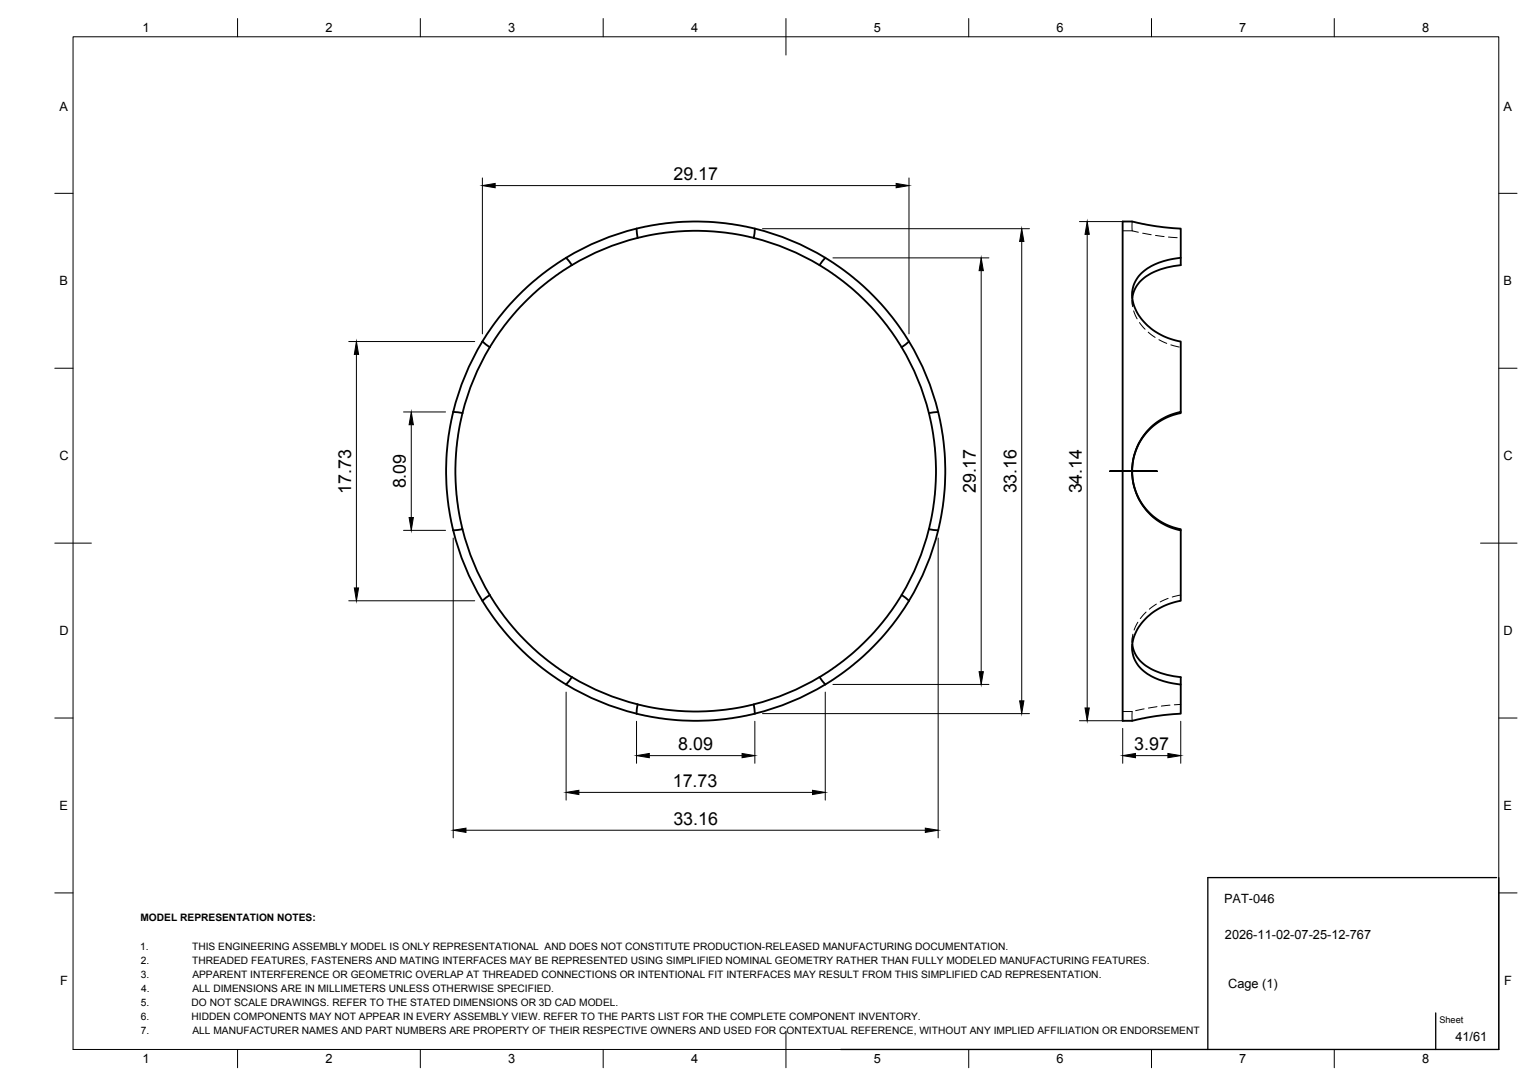
ISO-10303-21;
HEADER;
/* Generated by software containing ST-Developer
 * from STEP Tools, Inc. (www.steptools.com) 
 */

FILE_DESCRIPTION(
/* description */ ('Gear mesh backlash fixture'),
/* implementation_level */ '2;1');

FILE_NAME(
/* name */ 'Cage (1).step',
/* time_stamp */ '2026-10-28T03:26:00-07:00',
/* author */ (''),
/* organization */ (''),
/* preprocessor_version */ 'ST-DEVELOPER v20.2',
/* originating_system */ 'Autodesk Translation Framework v15.17.0.0',
/* authorisation */ '');

FILE_SCHEMA (('AUTOMOTIVE_DESIGN { 1 0 10303 214 3 1 1 }'));
ENDSEC;

DATA;
#10=MECHANICAL_DESIGN_GEOMETRIC_PRESENTATION_REPRESENTATION('',(#1061),#57900);
#751=SPHERICAL_SURFACE('',#14966,0.412776);
#752=SPHERICAL_SURFACE('',#14982,0.412776);
#753=SPHERICAL_SURFACE('',#14987,0.412776);
#754=SPHERICAL_SURFACE('',#14992,0.412776);
#755=SPHERICAL_SURFACE('',#14997,0.412776);
#756=SPHERICAL_SURFACE('',#15002,0.412776);
#757=SPHERICAL_SURFACE('',#15007,0.412776);
#758=SPHERICAL_SURFACE('',#15015,0.412776);
#809=B_SPLINE_CURVE_WITH_KNOTS('',3,(#21520,#21521,#21522,#21523,#21524,
#21525,#21526,#21527,#21528,#21529,#21530,#21531,#21532,#21533,#21534,#21535,
#21536,#21537,#21538,#21539,#21540,#21541),.UNSPECIFIED.,.F.,.F.,(4,2,2,
2,2,2,2,2,2,2,4),(0.0789094028588958,0.210573405340968,0.315860108011452,
0.421146810681936,0.522142632548711,0.623138454415485,0.72413427628226,
0.825130098149035,0.930416800819519,1.03570350349,1.16736750597208),
 .UNSPECIFIED.);
#810=B_SPLINE_CURVE_WITH_KNOTS('',3,(#21545,#21546,#21547,#21548,#21549,
#21550,#21551,#21552,#21553,#21554,#21555,#21556,#21557,#21558,#21559,#21560,
#21561,#21562,#21563,#21564,#21565,#21566),.UNSPECIFIED.,.F.,.F.,(4,2,2,
2,2,2,2,2,2,2,4),(0.0774793363974613,0.142088896491891,0.284177792983782,
0.411119756996526,0.514392970548519,0.617666184100513,0.720939397652506,
0.8242126112045,0.951154575217244,1.09324347170913,1.15785303180356),
 .UNSPECIFIED.);
#811=B_SPLINE_CURVE_WITH_KNOTS('',3,(#21572,#21573,#21574,#21575,#21576,
#21577,#21578,#21579,#21580,#21581,#21582,#21583,#21584,#21585,#21586,#21587,
#21588,#21589,#21590,#21591,#21592,#21593),.UNSPECIFIED.,.F.,.F.,(4,2,2,
2,2,2,2,2,2,2,4),(0.0774793363974613,0.142088896491891,0.284177792983782,
0.411119756996525,0.514392970548519,0.617666184100513,0.720939397652506,
0.8242126112045,0.951154575217243,1.09324347170913,1.15785303180356),
 .UNSPECIFIED.);
#812=B_SPLINE_CURVE_WITH_KNOTS('',3,(#21597,#21598,#21599,#21600,#21601,
#21602,#21603,#21604,#21605,#21606,#21607,#21608,#21609,#21610,#21611,#21612,
#21613,#21614,#21615,#21616,#21617,#21618),.UNSPECIFIED.,.F.,.F.,(4,2,2,
2,2,2,2,2,2,2,4),(0.0774793363974614,0.142088896491891,0.284177792983781,
0.411119756996525,0.514392970548519,0.617666184100512,0.720939397652506,
0.824212611204499,0.951154575217243,1.09324347170913,1.15785303180356),
 .UNSPECIFIED.);
#813=B_SPLINE_CURVE_WITH_KNOTS('',3,(#21622,#21623,#21624,#21625,#21626,
#21627,#21628,#21629,#21630,#21631,#21632,#21633),.UNSPECIFIED.,.F.,.F.,
(4,2,2,2,2,4),(0.0774793363974613,0.142088896491891,0.284177792983781,0.411119756996525,
0.514392970548519,0.617666184100512),.UNSPECIFIED.);
#814=B_SPLINE_CURVE_WITH_KNOTS('',3,(#21638,#21639,#21640,#21641,#21642,
#21643,#21644,#21645,#21646,#21647,#21648,#21649),.UNSPECIFIED.,.F.,.F.,
(4,2,2,2,2,4),(0.617666184100512,0.720939397652506,0.824212611204499,0.951154575217243,
1.09324347170913,1.15785303180356),.UNSPECIFIED.);
#815=B_SPLINE_CURVE_WITH_KNOTS('',3,(#21653,#21654,#21655,#21656,#21657,
#21658,#21659,#21660,#21661,#21662,#21663,#21664,#21665,#21666,#21667,#21668,
#21669,#21670,#21671,#21672,#21673,#21674),.UNSPECIFIED.,.F.,.F.,(4,2,2,
2,2,2,2,2,2,2,4),(0.0774793363974613,0.142088896491891,0.284177792983782,
0.411119756996526,0.514392970548519,0.617666184100513,0.720939397652507,
0.8242126112045,0.951154575217245,1.09324347170914,1.15785303180356),
 .UNSPECIFIED.);
#816=B_SPLINE_CURVE_WITH_KNOTS('',3,(#21678,#21679,#21680,#21681,#21682,
#21683,#21684,#21685,#21686,#21687,#21688,#21689,#21690,#21691,#21692,#21693,
#21694,#21695,#21696,#21697,#21698,#21699),.UNSPECIFIED.,.F.,.F.,(4,2,2,
2,2,2,2,2,2,2,4),(0.0774793363974613,0.142088896491891,0.284177792983782,
0.411119756996526,0.514392970548519,0.617666184100513,0.720939397652506,
0.824212611204499,0.951154575217243,1.09324347170913,1.15785303180356),
 .UNSPECIFIED.);
#817=B_SPLINE_CURVE_WITH_KNOTS('',3,(#21703,#21704,#21705,#21706,#21707,
#21708,#21709,#21710,#21711,#21712,#21713,#21714,#21715,#21716,#21717,#21718,
#21719,#21720,#21721,#21722,#21723,#21724),.UNSPECIFIED.,.F.,.F.,(4,2,2,
2,2,2,2,2,2,2,4),(0.0774793363974613,0.142088896491891,0.284177792983782,
0.411119756996526,0.514392970548519,0.617666184100513,0.720939397652506,
0.8242126112045,0.951154575217244,1.09324347170913,1.15785303180356),
 .UNSPECIFIED.);
#818=B_SPLINE_CURVE_WITH_KNOTS('',3,(#21728,#21729,#21730,#21731,#21732,
#21733,#21734,#21735,#21736,#21737,#21738,#21739,#21740,#21741,#21742,#21743,
#21744,#21745,#21746,#21747,#21748,#21749),.UNSPECIFIED.,.F.,.F.,(4,2,2,
2,2,2,2,2,2,2,4),(0.0774793363974613,0.142088896491891,0.284177792983782,
0.411119756996526,0.514392970548519,0.617666184100513,0.720939397652506,
0.8242126112045,0.951154575217243,1.09324347170913,1.15785303180356),
 .UNSPECIFIED.);
#819=B_SPLINE_CURVE_WITH_KNOTS('',3,(#21757,#21758,#21759,#21760,#21761,
#21762,#21763,#21764,#21765,#21766,#21767,#21768,#21769,#21770,#21771,#21772,
#21773,#21774,#21775,#21776,#21777,#21778),.UNSPECIFIED.,.F.,.F.,(4,2,2,
2,2,2,2,2,2,2,4),(0.0789094028588958,0.210573405340968,0.315860108011452,
0.421146810681936,0.522142632548711,0.623138454415485,0.72413427628226,
0.825130098149035,0.930416800819519,1.03570350349,1.16736750597208),
 .UNSPECIFIED.);
#820=B_SPLINE_CURVE_WITH_KNOTS('',3,(#21786,#21787,#21788,#21789,#21790,
#21791,#21792,#21793,#21794,#21795,#21796,#21797,#21798,#21799,#21800,#21801,
#21802,#21803,#21804,#21805,#21806,#21807),.UNSPECIFIED.,.F.,.F.,(4,2,2,
2,2,2,2,2,2,2,4),(0.0789094028588958,0.210573405340969,0.315860108011453,
0.421146810681937,0.522142632548712,0.623138454415486,0.724134276282261,
0.825130098149035,0.930416800819519,1.03570350349,1.16736750597208),
 .UNSPECIFIED.);
#821=B_SPLINE_CURVE_WITH_KNOTS('',3,(#21816,#21817,#21818,#21819,#21820,
#21821,#21822,#21823,#21824,#21825,#21826,#21827),.UNSPECIFIED.,.F.,.F.,
(4,2,2,2,2,4),(0.0789094028588958,0.210573405340968,0.315860108011452,0.421146810681937,
0.522142632548711,0.623138454415486),.UNSPECIFIED.);
#822=B_SPLINE_CURVE_WITH_KNOTS('',3,(#21829,#21830,#21831,#21832,#21833,
#21834,#21835,#21836,#21837,#21838,#21839,#21840),.UNSPECIFIED.,.F.,.F.,
(4,2,2,2,2,4),(0.623138454415486,0.72413427628226,0.825130098149035,0.930416800819519,
1.03570350349,1.16736750597208),.UNSPECIFIED.);
#823=B_SPLINE_CURVE_WITH_KNOTS('',3,(#21847,#21848,#21849,#21850,#21851,
#21852,#21853,#21854,#21855,#21856,#21857,#21858,#21859,#21860,#21861,#21862,
#21863,#21864,#21865,#21866,#21867,#21868),.UNSPECIFIED.,.F.,.F.,(4,2,2,
2,2,2,2,2,2,2,4),(0.0789094028588958,0.210573405340968,0.315860108011452,
0.421146810681936,0.522142632548711,0.623138454415486,0.72413427628226,
0.825130098149035,0.930416800819519,1.03570350349,1.16736750597208),
 .UNSPECIFIED.);
#824=B_SPLINE_CURVE_WITH_KNOTS('',3,(#21876,#21877,#21878,#21879,#21880,
#21881,#21882,#21883,#21884,#21885,#21886,#21887,#21888,#21889,#21890,#21891,
#21892,#21893,#21894,#21895,#21896,#21897),.UNSPECIFIED.,.F.,.F.,(4,2,2,
2,2,2,2,2,2,2,4),(0.0789094028588957,0.210573405340968,0.315860108011452,
0.421146810681936,0.522142632548711,0.623138454415485,0.72413427628226,
0.825130098149035,0.930416800819519,1.03570350349,1.16736750597207),
 .UNSPECIFIED.);
#825=B_SPLINE_CURVE_WITH_KNOTS('',3,(#21905,#21906,#21907,#21908,#21909,
#21910,#21911,#21912,#21913,#21914,#21915,#21916,#21917,#21918,#21919,#21920,
#21921,#21922,#21923,#21924,#21925,#21926),.UNSPECIFIED.,.F.,.F.,(4,2,2,
2,2,2,2,2,2,2,4),(0.0789094028588958,0.210573405340968,0.315860108011452,
0.421146810681936,0.522142632548711,0.623138454415486,0.72413427628226,
0.825130098149035,0.930416800819519,1.03570350349,1.16736750597208),
 .UNSPECIFIED.);
#826=B_SPLINE_CURVE_WITH_KNOTS('',3,(#21935,#21936,#21937,#21938,#21939,
#21940,#21941,#21942,#21943,#21944,#21945,#21946,#21947,#21948,#21949,#21950,
#21951,#21952,#21953,#21954,#21955,#21956),.UNSPECIFIED.,.F.,.F.,(4,2,2,
2,2,2,2,2,2,2,4),(0.0789094028588958,0.210573405340968,0.315860108011452,
0.421146810681936,0.522142632548711,0.623138454415485,0.72413427628226,
0.825130098149035,0.930416800819519,1.03570350349,1.16736750597208),
 .UNSPECIFIED.);
#947=SHAPE_REPRESENTATION_RELATIONSHIP('SRR','None',#58146,#997);
#997=ADVANCED_BREP_SHAPE_REPRESENTATION('',(#1124),#57879);
#1061=STYLED_ITEM('',(#58465),#1124);
#1124=MANIFOLD_SOLID_BREP('Continuous crown cage',#13623);
#1286=FACE_BOUND('',#2994,.T.);
#1536=PLANE('',#14979);
#1537=PLANE('',#14984);
#1538=PLANE('',#14989);
#1539=PLANE('',#14994);
#1540=PLANE('',#14999);
#1541=PLANE('',#15004);
#1542=PLANE('',#15013);
#1543=PLANE('',#15017);
#1544=PLANE('',#15018);
#2068=FACE_OUTER_BOUND('',#2976,.T.);
#2069=FACE_OUTER_BOUND('',#2977,.T.);
#2070=FACE_OUTER_BOUND('',#2978,.T.);
#2071=FACE_OUTER_BOUND('',#2979,.T.);
#2072=FACE_OUTER_BOUND('',#2980,.T.);
#2073=FACE_OUTER_BOUND('',#2981,.T.);
#2074=FACE_OUTER_BOUND('',#2982,.T.);
#2075=FACE_OUTER_BOUND('',#2983,.T.);
#2076=FACE_OUTER_BOUND('',#2984,.T.);
#2077=FACE_OUTER_BOUND('',#2985,.T.);
#2078=FACE_OUTER_BOUND('',#2986,.T.);
#2079=FACE_OUTER_BOUND('',#2987,.T.);
#2080=FACE_OUTER_BOUND('',#2988,.T.);
#2081=FACE_OUTER_BOUND('',#2989,.T.);
#2082=FACE_OUTER_BOUND('',#2990,.T.);
#2083=FACE_OUTER_BOUND('',#2991,.T.);
#2084=FACE_OUTER_BOUND('',#2992,.T.);
#2085=FACE_OUTER_BOUND('',#2993,.T.);
#2086=FACE_OUTER_BOUND('',#2995,.T.);
#2976=EDGE_LOOP('',(#10555,#10556,#10557,#10558));
#2977=EDGE_LOOP('',(#10559,#10560,#10561,#10562,#10563,#10564,#10565,#10566,
#10567,#10568,#10569,#10570,#10571,#10572,#10573,#10574,#10575,#10576,#10577,
#10578));
#2978=EDGE_LOOP('',(#10579,#10580,#10581,#10582));
#2979=EDGE_LOOP('',(#10583,#10584,#10585,#10586));
#2980=EDGE_LOOP('',(#10587,#10588,#10589,#10590));
#2981=EDGE_LOOP('',(#10591,#10592,#10593,#10594));
#2982=EDGE_LOOP('',(#10595,#10596,#10597,#10598));
#2983=EDGE_LOOP('',(#10599,#10600,#10601,#10602,#10603,#10604));
#2984=EDGE_LOOP('',(#10605,#10606,#10607,#10608));
#2985=EDGE_LOOP('',(#10609,#10610,#10611,#10612));
#2986=EDGE_LOOP('',(#10613,#10614,#10615,#10616));
#2987=EDGE_LOOP('',(#10617,#10618,#10619,#10620));
#2988=EDGE_LOOP('',(#10621,#10622,#10623,#10624));
#2989=EDGE_LOOP('',(#10625,#10626,#10627,#10628));
#2990=EDGE_LOOP('',(#10629,#10630,#10631,#10632,#10633,#10634,#10635,#10636,
#10637,#10638,#10639,#10640,#10641,#10642,#10643,#10644,#10645,#10646,#10647,
#10648));
#2991=EDGE_LOOP('',(#10649,#10650,#10651,#10652));
#2992=EDGE_LOOP('',(#10653,#10654,#10655,#10656));
#2993=EDGE_LOOP('',(#10657));
#2994=EDGE_LOOP('',(#10658));
#2995=EDGE_LOOP('',(#10659,#10660,#10661,#10662));
#3873=LINE('',#21635,#4762);
#3874=LINE('',#21931,#4763);
#4762=VECTOR('',#17596,1.706752);
#4763=VECTOR('',#17673,1.643248);
#5540=CIRCLE('',#14967,0.405071403305639);
#5541=CIRCLE('',#14968,0.405071403305639);
#5542=CIRCLE('',#14970,1.706752);
#5543=CIRCLE('',#14971,1.706752);
#5544=CIRCLE('',#14972,1.706752);
#5545=CIRCLE('',#14973,1.706752);
#5546=CIRCLE('',#14974,1.706752);
#5547=CIRCLE('',#14975,1.706752);
#5548=CIRCLE('',#14976,1.706752);
#5549=CIRCLE('',#14977,1.706752);
#5550=CIRCLE('',#14978,1.706752);
#5551=CIRCLE('',#14980,1.643248);
#5552=CIRCLE('',#14981,0.405071403305639);
#5553=CIRCLE('',#14983,0.405071403305639);
#5554=CIRCLE('',#14985,1.643248);
#5555=CIRCLE('',#14986,0.405071403305639);
#5556=CIRCLE('',#14988,0.405071403305639);
#5557=CIRCLE('',#14990,1.643248);
#5558=CIRCLE('',#14991,0.405071403305639);
#5559=CIRCLE('',#14993,0.405071403305639);
#5560=CIRCLE('',#14995,1.643248);
#5561=CIRCLE('',#14996,0.405071403305639);
#5562=CIRCLE('',#14998,0.405071403305639);
#5563=CIRCLE('',#15000,1.643248);
#5564=CIRCLE('',#15001,0.405071403305639);
#5565=CIRCLE('',#15003,0.405071403305639);
#5566=CIRCLE('',#15005,1.643248);
#5567=CIRCLE('',#15006,0.405071403305639);
#5568=CIRCLE('',#15008,0.405071403305639);
#5569=CIRCLE('',#15010,1.643248);
#5570=CIRCLE('',#15011,1.643248);
#5571=CIRCLE('',#15012,1.643248);
#5572=CIRCLE('',#15014,0.405071403305639);
#5573=CIRCLE('',#15016,0.405071403305639);
#6350=VERTEX_POINT('',#21518);
#6351=VERTEX_POINT('',#21519);
#6352=VERTEX_POINT('',#21542);
#6353=VERTEX_POINT('',#21544);
#6354=VERTEX_POINT('',#21569);
#6355=VERTEX_POINT('',#21571);
#6356=VERTEX_POINT('',#21594);
#6357=VERTEX_POINT('',#21596);
#6358=VERTEX_POINT('',#21619);
#6359=VERTEX_POINT('',#21621);
#6360=VERTEX_POINT('',#21634);
#6361=VERTEX_POINT('',#21637);
#6362=VERTEX_POINT('',#21650);
#6363=VERTEX_POINT('',#21652);
#6364=VERTEX_POINT('',#21675);
#6365=VERTEX_POINT('',#21677);
#6366=VERTEX_POINT('',#21700);
#6367=VERTEX_POINT('',#21702);
#6368=VERTEX_POINT('',#21725);
#6369=VERTEX_POINT('',#21727);
#6370=VERTEX_POINT('',#21752);
#6371=VERTEX_POINT('',#21756);
#6372=VERTEX_POINT('',#21781);
#6373=VERTEX_POINT('',#21785);
#6374=VERTEX_POINT('',#21810);
#6375=VERTEX_POINT('',#21814);
#6376=VERTEX_POINT('',#21815);
#6377=VERTEX_POINT('',#21842);
#6378=VERTEX_POINT('',#21846);
#6379=VERTEX_POINT('',#21871);
#6380=VERTEX_POINT('',#21875);
#6381=VERTEX_POINT('',#21900);
#6382=VERTEX_POINT('',#21904);
#6383=VERTEX_POINT('',#21929);
#6384=VERTEX_POINT('',#21932);
#6385=VERTEX_POINT('',#21934);
#7864=EDGE_CURVE('',#6350,#6351,#809,.T.);
#7865=EDGE_CURVE('',#6352,#6350,#5540,.T.);
#7866=EDGE_CURVE('',#6353,#6352,#810,.T.);
#7867=EDGE_CURVE('',#6351,#6353,#5541,.T.);
#7868=EDGE_CURVE('',#6354,#6352,#5542,.T.);
#7869=EDGE_CURVE('',#6354,#6355,#811,.T.);
#7870=EDGE_CURVE('',#6356,#6355,#5543,.T.);
#7871=EDGE_CURVE('',#6356,#6357,#812,.T.);
#7872=EDGE_CURVE('',#6358,#6357,#5544,.T.);
#7873=EDGE_CURVE('',#6358,#6359,#813,.T.);
#7874=EDGE_CURVE('',#6359,#6360,#3873,.T.);
#7875=EDGE_CURVE('',#6360,#6360,#5545,.T.);
#7876=EDGE_CURVE('',#6359,#6361,#814,.T.);
#7877=EDGE_CURVE('',#6362,#6361,#5546,.T.);
#7878=EDGE_CURVE('',#6362,#6363,#815,.T.);
#7879=EDGE_CURVE('',#6364,#6363,#5547,.T.);
#7880=EDGE_CURVE('',#6364,#6365,#816,.T.);
#7881=EDGE_CURVE('',#6366,#6365,#5548,.T.);
#7882=EDGE_CURVE('',#6366,#6367,#817,.T.);
#7883=EDGE_CURVE('',#6368,#6367,#5549,.T.);
#7884=EDGE_CURVE('',#6368,#6369,#818,.T.);
#7885=EDGE_CURVE('',#6353,#6369,#5550,.T.);
#7886=EDGE_CURVE('',#6350,#6370,#5551,.T.);
#7887=EDGE_CURVE('',#6370,#6354,#5552,.T.);
#7888=EDGE_CURVE('',#6371,#6370,#819,.T.);
#7889=EDGE_CURVE('',#6355,#6371,#5553,.T.);
#7890=EDGE_CURVE('',#6371,#6372,#5554,.T.);
#7891=EDGE_CURVE('',#6372,#6356,#5555,.T.);
#7892=EDGE_CURVE('',#6373,#6372,#820,.T.);
#7893=EDGE_CURVE('',#6357,#6373,#5556,.T.);
#7894=EDGE_CURVE('',#6373,#6374,#5557,.T.);
#7895=EDGE_CURVE('',#6374,#6358,#5558,.T.);
#7896=EDGE_CURVE('',#6375,#6376,#821,.T.);
#7897=EDGE_CURVE('',#6361,#6375,#5559,.T.);
#7898=EDGE_CURVE('',#6376,#6374,#822,.T.);
#7899=EDGE_CURVE('',#6375,#6377,#5560,.T.);
#7900=EDGE_CURVE('',#6377,#6362,#5561,.T.);
#7901=EDGE_CURVE('',#6378,#6377,#823,.T.);
#7902=EDGE_CURVE('',#6363,#6378,#5562,.T.);
#7903=EDGE_CURVE('',#6378,#6379,#5563,.T.);
#7904=EDGE_CURVE('',#6379,#6364,#5564,.T.);
#7905=EDGE_CURVE('',#6380,#6379,#824,.T.);
#7906=EDGE_CURVE('',#6365,#6380,#5565,.T.);
#7907=EDGE_CURVE('',#6380,#6381,#5566,.T.);
#7908=EDGE_CURVE('',#6381,#6366,#5567,.T.);
#7909=EDGE_CURVE('',#6382,#6381,#825,.T.);
#7910=EDGE_CURVE('',#6367,#6382,#5568,.T.);
#7911=EDGE_CURVE('',#6383,#6383,#5569,.T.);
#7912=EDGE_CURVE('',#6383,#6376,#3874,.T.);
#7913=EDGE_CURVE('',#6384,#6351,#5570,.T.);
#7914=EDGE_CURVE('',#6384,#6385,#826,.T.);
#7915=EDGE_CURVE('',#6382,#6385,#5571,.T.);
#7916=EDGE_CURVE('',#6369,#6384,#5572,.T.);
#7917=EDGE_CURVE('',#6385,#6368,#5573,.T.);
#10555=ORIENTED_EDGE('',*,*,#7864,.F.);
#10556=ORIENTED_EDGE('',*,*,#7865,.F.);
#10557=ORIENTED_EDGE('',*,*,#7866,.F.);
#10558=ORIENTED_EDGE('',*,*,#7867,.F.);
#10559=ORIENTED_EDGE('',*,*,#7866,.T.);
#10560=ORIENTED_EDGE('',*,*,#7868,.F.);
#10561=ORIENTED_EDGE('',*,*,#7869,.T.);
#10562=ORIENTED_EDGE('',*,*,#7870,.F.);
#10563=ORIENTED_EDGE('',*,*,#7871,.T.);
#10564=ORIENTED_EDGE('',*,*,#7872,.F.);
#10565=ORIENTED_EDGE('',*,*,#7873,.T.);
#10566=ORIENTED_EDGE('',*,*,#7874,.T.);
#10567=ORIENTED_EDGE('',*,*,#7875,.F.);
#10568=ORIENTED_EDGE('',*,*,#7874,.F.);
#10569=ORIENTED_EDGE('',*,*,#7876,.T.);
#10570=ORIENTED_EDGE('',*,*,#7877,.F.);
#10571=ORIENTED_EDGE('',*,*,#7878,.T.);
#10572=ORIENTED_EDGE('',*,*,#7879,.F.);
#10573=ORIENTED_EDGE('',*,*,#7880,.T.);
#10574=ORIENTED_EDGE('',*,*,#7881,.F.);
#10575=ORIENTED_EDGE('',*,*,#7882,.T.);
#10576=ORIENTED_EDGE('',*,*,#7883,.F.);
#10577=ORIENTED_EDGE('',*,*,#7884,.T.);
#10578=ORIENTED_EDGE('',*,*,#7885,.F.);
#10579=ORIENTED_EDGE('',*,*,#7865,.T.);
#10580=ORIENTED_EDGE('',*,*,#7886,.T.);
#10581=ORIENTED_EDGE('',*,*,#7887,.T.);
#10582=ORIENTED_EDGE('',*,*,#7868,.T.);
#10583=ORIENTED_EDGE('',*,*,#7888,.F.);
#10584=ORIENTED_EDGE('',*,*,#7889,.F.);
#10585=ORIENTED_EDGE('',*,*,#7869,.F.);
#10586=ORIENTED_EDGE('',*,*,#7887,.F.);
#10587=ORIENTED_EDGE('',*,*,#7889,.T.);
#10588=ORIENTED_EDGE('',*,*,#7890,.T.);
#10589=ORIENTED_EDGE('',*,*,#7891,.T.);
#10590=ORIENTED_EDGE('',*,*,#7870,.T.);
#10591=ORIENTED_EDGE('',*,*,#7892,.F.);
#10592=ORIENTED_EDGE('',*,*,#7893,.F.);
#10593=ORIENTED_EDGE('',*,*,#7871,.F.);
#10594=ORIENTED_EDGE('',*,*,#7891,.F.);
#10595=ORIENTED_EDGE('',*,*,#7893,.T.);
#10596=ORIENTED_EDGE('',*,*,#7894,.T.);
#10597=ORIENTED_EDGE('',*,*,#7895,.T.);
#10598=ORIENTED_EDGE('',*,*,#7872,.T.);
#10599=ORIENTED_EDGE('',*,*,#7896,.F.);
#10600=ORIENTED_EDGE('',*,*,#7897,.F.);
#10601=ORIENTED_EDGE('',*,*,#7876,.F.);
#10602=ORIENTED_EDGE('',*,*,#7873,.F.);
#10603=ORIENTED_EDGE('',*,*,#7895,.F.);
#10604=ORIENTED_EDGE('',*,*,#7898,.F.);
#10605=ORIENTED_EDGE('',*,*,#7897,.T.);
#10606=ORIENTED_EDGE('',*,*,#7899,.T.);
#10607=ORIENTED_EDGE('',*,*,#7900,.T.);
#10608=ORIENTED_EDGE('',*,*,#7877,.T.);
#10609=ORIENTED_EDGE('',*,*,#7901,.F.);
#10610=ORIENTED_EDGE('',*,*,#7902,.F.);
#10611=ORIENTED_EDGE('',*,*,#7878,.F.);
#10612=ORIENTED_EDGE('',*,*,#7900,.F.);
#10613=ORIENTED_EDGE('',*,*,#7902,.T.);
#10614=ORIENTED_EDGE('',*,*,#7903,.T.);
#10615=ORIENTED_EDGE('',*,*,#7904,.T.);
#10616=ORIENTED_EDGE('',*,*,#7879,.T.);
#10617=ORIENTED_EDGE('',*,*,#7905,.F.);
#10618=ORIENTED_EDGE('',*,*,#7906,.F.);
#10619=ORIENTED_EDGE('',*,*,#7880,.F.);
#10620=ORIENTED_EDGE('',*,*,#7904,.F.);
#10621=ORIENTED_EDGE('',*,*,#7906,.T.);
#10622=ORIENTED_EDGE('',*,*,#7907,.T.);
#10623=ORIENTED_EDGE('',*,*,#7908,.T.);
#10624=ORIENTED_EDGE('',*,*,#7881,.T.);
#10625=ORIENTED_EDGE('',*,*,#7882,.F.);
#10626=ORIENTED_EDGE('',*,*,#7908,.F.);
#10627=ORIENTED_EDGE('',*,*,#7909,.F.);
#10628=ORIENTED_EDGE('',*,*,#7910,.F.);
#10629=ORIENTED_EDGE('',*,*,#7911,.F.);
#10630=ORIENTED_EDGE('',*,*,#7912,.T.);
#10631=ORIENTED_EDGE('',*,*,#7898,.T.);
#10632=ORIENTED_EDGE('',*,*,#7894,.F.);
#10633=ORIENTED_EDGE('',*,*,#7892,.T.);
#10634=ORIENTED_EDGE('',*,*,#7890,.F.);
#10635=ORIENTED_EDGE('',*,*,#7888,.T.);
#10636=ORIENTED_EDGE('',*,*,#7886,.F.);
#10637=ORIENTED_EDGE('',*,*,#7864,.T.);
#10638=ORIENTED_EDGE('',*,*,#7913,.F.);
#10639=ORIENTED_EDGE('',*,*,#7914,.T.);
#10640=ORIENTED_EDGE('',*,*,#7915,.F.);
#10641=ORIENTED_EDGE('',*,*,#7909,.T.);
#10642=ORIENTED_EDGE('',*,*,#7907,.F.);
#10643=ORIENTED_EDGE('',*,*,#7905,.T.);
#10644=ORIENTED_EDGE('',*,*,#7903,.F.);
#10645=ORIENTED_EDGE('',*,*,#7901,.T.);
#10646=ORIENTED_EDGE('',*,*,#7899,.F.);
#10647=ORIENTED_EDGE('',*,*,#7896,.T.);
#10648=ORIENTED_EDGE('',*,*,#7912,.F.);
#10649=ORIENTED_EDGE('',*,*,#7867,.T.);
#10650=ORIENTED_EDGE('',*,*,#7885,.T.);
#10651=ORIENTED_EDGE('',*,*,#7916,.T.);
#10652=ORIENTED_EDGE('',*,*,#7913,.T.);
#10653=ORIENTED_EDGE('',*,*,#7884,.F.);
#10654=ORIENTED_EDGE('',*,*,#7917,.F.);
#10655=ORIENTED_EDGE('',*,*,#7914,.F.);
#10656=ORIENTED_EDGE('',*,*,#7916,.F.);
#10657=ORIENTED_EDGE('',*,*,#7875,.T.);
#10658=ORIENTED_EDGE('',*,*,#7911,.T.);
#10659=ORIENTED_EDGE('',*,*,#7910,.T.);
#10660=ORIENTED_EDGE('',*,*,#7915,.T.);
#10661=ORIENTED_EDGE('',*,*,#7917,.T.);
#10662=ORIENTED_EDGE('',*,*,#7883,.T.);
#12710=CYLINDRICAL_SURFACE('',#14969,1.706752);
#12711=CYLINDRICAL_SURFACE('',#15009,1.643248);
#13185=ADVANCED_FACE('',(#2068),#751,.F.);
#13186=ADVANCED_FACE('',(#2069),#12710,.T.);
#13187=ADVANCED_FACE('',(#2070),#1536,.T.);
#13188=ADVANCED_FACE('',(#2071),#752,.F.);
#13189=ADVANCED_FACE('',(#2072),#1537,.T.);
#13190=ADVANCED_FACE('',(#2073),#753,.F.);
#13191=ADVANCED_FACE('',(#2074),#1538,.T.);
#13192=ADVANCED_FACE('',(#2075),#754,.F.);
#13193=ADVANCED_FACE('',(#2076),#1539,.T.);
#13194=ADVANCED_FACE('',(#2077),#755,.F.);
#13195=ADVANCED_FACE('',(#2078),#1540,.T.);
#13196=ADVANCED_FACE('',(#2079),#756,.F.);
#13197=ADVANCED_FACE('',(#2080),#1541,.T.);
#13198=ADVANCED_FACE('',(#2081),#757,.F.);
#13199=ADVANCED_FACE('',(#2082),#12711,.F.);
#13200=ADVANCED_FACE('',(#2083),#1542,.T.);
#13201=ADVANCED_FACE('',(#2084),#758,.F.);
#13202=ADVANCED_FACE('',(#2085,#1286),#1543,.T.);
#13203=ADVANCED_FACE('',(#2086),#1544,.T.);
#13623=CLOSED_SHELL('',(#13185,#13186,#13187,#13188,#13189,#13190,#13191,
#13192,#13193,#13194,#13195,#13196,#13197,#13198,#13199,#13200,#13201,#13202,
#13203));
#14965=AXIS2_PLACEMENT_3D('',#21516,#17580,#17581);
#14966=AXIS2_PLACEMENT_3D('',#21517,#17582,#17583);
#14967=AXIS2_PLACEMENT_3D('',#21543,#17584,#17585);
#14968=AXIS2_PLACEMENT_3D('',#21567,#17586,#17587);
#14969=AXIS2_PLACEMENT_3D('',#21568,#17588,#17589);
#14970=AXIS2_PLACEMENT_3D('',#21570,#17590,#17591);
#14971=AXIS2_PLACEMENT_3D('',#21595,#17592,#17593);
#14972=AXIS2_PLACEMENT_3D('',#21620,#17594,#17595);
#14973=AXIS2_PLACEMENT_3D('',#21636,#17597,#17598);
#14974=AXIS2_PLACEMENT_3D('',#21651,#17599,#17600);
#14975=AXIS2_PLACEMENT_3D('',#21676,#17601,#17602);
#14976=AXIS2_PLACEMENT_3D('',#21701,#17603,#17604);
#14977=AXIS2_PLACEMENT_3D('',#21726,#17605,#17606);
#14978=AXIS2_PLACEMENT_3D('',#21750,#17607,#17608);
#14979=AXIS2_PLACEMENT_3D('',#21751,#17609,#17610);
#14980=AXIS2_PLACEMENT_3D('',#21753,#17611,#17612);
#14981=AXIS2_PLACEMENT_3D('',#21754,#17613,#17614);
#14982=AXIS2_PLACEMENT_3D('',#21755,#17615,#17616);
#14983=AXIS2_PLACEMENT_3D('',#21779,#17617,#17618);
#14984=AXIS2_PLACEMENT_3D('',#21780,#17619,#17620);
#14985=AXIS2_PLACEMENT_3D('',#21782,#17621,#17622);
#14986=AXIS2_PLACEMENT_3D('',#21783,#17623,#17624);
#14987=AXIS2_PLACEMENT_3D('',#21784,#17625,#17626);
#14988=AXIS2_PLACEMENT_3D('',#21808,#17627,#17628);
#14989=AXIS2_PLACEMENT_3D('',#21809,#17629,#17630);
#14990=AXIS2_PLACEMENT_3D('',#21811,#17631,#17632);
#14991=AXIS2_PLACEMENT_3D('',#21812,#17633,#17634);
#14992=AXIS2_PLACEMENT_3D('',#21813,#17635,#17636);
#14993=AXIS2_PLACEMENT_3D('',#21828,#17637,#17638);
#14994=AXIS2_PLACEMENT_3D('',#21841,#17639,#17640);
#14995=AXIS2_PLACEMENT_3D('',#21843,#17641,#17642);
#14996=AXIS2_PLACEMENT_3D('',#21844,#17643,#17644);
#14997=AXIS2_PLACEMENT_3D('',#21845,#17645,#17646);
#14998=AXIS2_PLACEMENT_3D('',#21869,#17647,#17648);
#14999=AXIS2_PLACEMENT_3D('',#21870,#17649,#17650);
#15000=AXIS2_PLACEMENT_3D('',#21872,#17651,#17652);
#15001=AXIS2_PLACEMENT_3D('',#21873,#17653,#17654);
#15002=AXIS2_PLACEMENT_3D('',#21874,#17655,#17656);
#15003=AXIS2_PLACEMENT_3D('',#21898,#17657,#17658);
#15004=AXIS2_PLACEMENT_3D('',#21899,#17659,#17660);
#15005=AXIS2_PLACEMENT_3D('',#21901,#17661,#17662);
#15006=AXIS2_PLACEMENT_3D('',#21902,#17663,#17664);
#15007=AXIS2_PLACEMENT_3D('',#21903,#17665,#17666);
#15008=AXIS2_PLACEMENT_3D('',#21927,#17667,#17668);
#15009=AXIS2_PLACEMENT_3D('',#21928,#17669,#17670);
#15010=AXIS2_PLACEMENT_3D('',#21930,#17671,#17672);
#15011=AXIS2_PLACEMENT_3D('',#21933,#17674,#17675);
#15012=AXIS2_PLACEMENT_3D('',#21957,#17676,#17677);
#15013=AXIS2_PLACEMENT_3D('',#21958,#17678,#17679);
#15014=AXIS2_PLACEMENT_3D('',#21959,#17680,#17681);
#15015=AXIS2_PLACEMENT_3D('',#21960,#17682,#17683);
#15016=AXIS2_PLACEMENT_3D('',#21961,#17684,#17685);
#15017=AXIS2_PLACEMENT_3D('',#21962,#17686,#17687);
#15018=AXIS2_PLACEMENT_3D('',#21963,#17688,#17689);
#17580=DIRECTION('axis',(0.,0.,1.));
#17581=DIRECTION('refdir',(1.,0.,0.));
#17582=DIRECTION('center_axis',(0.,0.,1.));
#17583=DIRECTION('ref_axis',(1.,0.,0.));
#17584=DIRECTION('center_axis',(0.,-1.,0.));
#17585=DIRECTION('ref_axis',(0.,0.,-1.));
#17586=DIRECTION('center_axis',(0.,-1.,0.));
#17587=DIRECTION('ref_axis',(0.,0.,-1.));
#17588=DIRECTION('center_axis',(0.,1.,0.));
#17589=DIRECTION('ref_axis',(1.,0.,0.));
#17590=DIRECTION('center_axis',(0.,1.,0.));
#17591=DIRECTION('ref_axis',(1.,0.,0.));
#17592=DIRECTION('center_axis',(0.,1.,0.));
#17593=DIRECTION('ref_axis',(1.,0.,0.));
#17594=DIRECTION('center_axis',(0.,1.,0.));
#17595=DIRECTION('ref_axis',(1.,0.,0.));
#17596=DIRECTION('',(0.,-1.,0.));
#17597=DIRECTION('center_axis',(0.,-1.,0.));
#17598=DIRECTION('ref_axis',(1.,0.,0.));
#17599=DIRECTION('center_axis',(0.,1.,0.));
#17600=DIRECTION('ref_axis',(1.,0.,0.));
#17601=DIRECTION('center_axis',(0.,1.,0.));
#17602=DIRECTION('ref_axis',(1.,0.,0.));
#17603=DIRECTION('center_axis',(0.,1.,0.));
#17604=DIRECTION('ref_axis',(1.,0.,0.));
#17605=DIRECTION('center_axis',(0.,1.,0.));
#17606=DIRECTION('ref_axis',(1.,0.,0.));
#17607=DIRECTION('center_axis',(0.,1.,0.));
#17608=DIRECTION('ref_axis',(1.,0.,0.));
#17609=DIRECTION('center_axis',(0.,1.,0.));
#17610=DIRECTION('ref_axis',(1.,0.,0.));
#17611=DIRECTION('center_axis',(0.,-1.,0.));
#17612=DIRECTION('ref_axis',(1.,0.,0.));
#17613=DIRECTION('center_axis',(0.,-1.,0.));
#17614=DIRECTION('ref_axis',(0.,0.,-1.));
#17615=DIRECTION('center_axis',(6.12323399573677E-17,0.,1.));
#17616=DIRECTION('ref_axis',(1.,0.,0.));
#17617=DIRECTION('center_axis',(0.,-1.,0.));
#17618=DIRECTION('ref_axis',(0.,0.,-1.));
#17619=DIRECTION('center_axis',(0.,1.,0.));
#17620=DIRECTION('ref_axis',(1.,0.,0.));
#17621=DIRECTION('center_axis',(0.,-1.,0.));
#17622=DIRECTION('ref_axis',(1.,0.,0.));
#17623=DIRECTION('center_axis',(0.,-1.,0.));
#17624=DIRECTION('ref_axis',(0.,0.,-1.));
#17625=DIRECTION('center_axis',(0.,0.,1.));
#17626=DIRECTION('ref_axis',(1.,0.,0.));
#17627=DIRECTION('center_axis',(0.,-1.,0.));
#17628=DIRECTION('ref_axis',(0.,0.,-1.));
#17629=DIRECTION('center_axis',(0.,1.,0.));
#17630=DIRECTION('ref_axis',(1.,0.,0.));
#17631=DIRECTION('center_axis',(0.,-1.,0.));
#17632=DIRECTION('ref_axis',(1.,0.,0.));
#17633=DIRECTION('center_axis',(0.,-1.,0.));
#17634=DIRECTION('ref_axis',(0.,0.,-1.));
#17635=DIRECTION('center_axis',(0.,0.,1.));
#17636=DIRECTION('ref_axis',(1.,0.,0.));
#17637=DIRECTION('center_axis',(0.,-1.,0.));
#17638=DIRECTION('ref_axis',(0.,0.,-1.));
#17639=DIRECTION('center_axis',(0.,1.,0.));
#17640=DIRECTION('ref_axis',(1.,0.,0.));
#17641=DIRECTION('center_axis',(0.,-1.,0.));
#17642=DIRECTION('ref_axis',(1.,0.,0.));
#17643=DIRECTION('center_axis',(0.,-1.,0.));
#17644=DIRECTION('ref_axis',(0.,0.,-1.));
#17645=DIRECTION('center_axis',(0.,0.,1.));
#17646=DIRECTION('ref_axis',(1.,0.,0.));
#17647=DIRECTION('center_axis',(0.,-1.,0.));
#17648=DIRECTION('ref_axis',(0.,0.,-1.));
#17649=DIRECTION('center_axis',(0.,1.,0.));
#17650=DIRECTION('ref_axis',(1.,0.,0.));
#17651=DIRECTION('center_axis',(0.,-1.,0.));
#17652=DIRECTION('ref_axis',(1.,0.,0.));
#17653=DIRECTION('center_axis',(0.,-1.,0.));
#17654=DIRECTION('ref_axis',(0.,0.,-1.));
#17655=DIRECTION('center_axis',(6.12323399573676E-17,0.,1.));
#17656=DIRECTION('ref_axis',(1.,0.,0.));
#17657=DIRECTION('center_axis',(0.,-1.,0.));
#17658=DIRECTION('ref_axis',(0.,0.,-1.));
#17659=DIRECTION('center_axis',(0.,1.,0.));
#17660=DIRECTION('ref_axis',(1.,0.,0.));
#17661=DIRECTION('center_axis',(0.,-1.,0.));
#17662=DIRECTION('ref_axis',(1.,0.,0.));
#17663=DIRECTION('center_axis',(0.,-1.,0.));
#17664=DIRECTION('ref_axis',(0.,0.,-1.));
#17665=DIRECTION('center_axis',(0.,0.,1.));
#17666=DIRECTION('ref_axis',(1.,0.,0.));
#17667=DIRECTION('center_axis',(0.,-1.,0.));
#17668=DIRECTION('ref_axis',(0.,0.,-1.));
#17669=DIRECTION('center_axis',(0.,1.,0.));
#17670=DIRECTION('ref_axis',(1.,0.,0.));
#17671=DIRECTION('center_axis',(0.,1.,0.));
#17672=DIRECTION('ref_axis',(1.,0.,0.));
#17673=DIRECTION('',(0.,1.,0.));
#17674=DIRECTION('center_axis',(0.,-1.,0.));
#17675=DIRECTION('ref_axis',(1.,0.,0.));
#17676=DIRECTION('center_axis',(0.,-1.,0.));
#17677=DIRECTION('ref_axis',(1.,0.,0.));
#17678=DIRECTION('center_axis',(0.,1.,0.));
#17679=DIRECTION('ref_axis',(1.,0.,0.));
#17680=DIRECTION('center_axis',(0.,-1.,0.));
#17681=DIRECTION('ref_axis',(0.,0.,-1.));
#17682=DIRECTION('center_axis',(0.,0.,1.));
#17683=DIRECTION('ref_axis',(1.,0.,0.));
#17684=DIRECTION('center_axis',(0.,-1.,0.));
#17685=DIRECTION('ref_axis',(0.,0.,-1.));
#17686=DIRECTION('center_axis',(0.,-1.,0.));
#17687=DIRECTION('ref_axis',(-1.,0.,0.));
#17688=DIRECTION('center_axis',(0.,1.,0.));
#17689=DIRECTION('ref_axis',(1.,0.,0.));
#21516=CARTESIAN_POINT('',(0.,0.,0.));
#21517=CARTESIAN_POINT('Origin',(1.18440385848747,0.,1.18440385848747));
#21518=CARTESIAN_POINT('',(0.846804978391753,-0.07938,1.40825612658882));
#21519=CARTESIAN_POINT('',(1.40825612658882,-0.07938,0.846804978391754));
#21520=CARTESIAN_POINT('Ctrl Pts',(0.846804978391752,-0.0793800000000001,
1.40825612658882));
#21521=CARTESIAN_POINT('Ctrl Pts',(0.854205272175554,-0.123401821157026,
1.40380622184538));
#21522=CARTESIAN_POINT('Ctrl Pts',(0.867957148219441,-0.166543350814306,
1.39550172959303));
#21523=CARTESIAN_POINT('Ctrl Pts',(0.902193646979982,-0.237231147975234,
1.3735491215176));
#21524=CARTESIAN_POINT('Ctrl Pts',(0.920778333482564,-0.266264900654909,
1.36127834356734));
#21525=CARTESIAN_POINT('Ctrl Pts',(0.962485392528369,-0.317195968905306,
1.33211611256184));
#21526=CARTESIAN_POINT('Ctrl Pts',(0.985600426557816,-0.33909093068465,
1.31521005565926));
#21527=CARTESIAN_POINT('Ctrl Pts',(1.03253285680459,-0.373586846396559,
1.27866649102984));
#21528=CARTESIAN_POINT('Ctrl Pts',(1.05871835910697,-0.388086240756494,
1.25722555095714));
#21529=CARTESIAN_POINT('Ctrl Pts',(1.11153475808518,-0.407068917407805,
1.2107812086231));
#21530=CARTESIAN_POINT('Ctrl Pts',(1.13814686046673,-0.411552957311693,
1.18575674747573));
#21531=CARTESIAN_POINT('Ctrl Pts',(1.18575674747573,-0.411552957311693,
1.13814686046673));
#21532=CARTESIAN_POINT('Ctrl Pts',(1.2107812086231,-0.407068917407805,1.11153475808518));
#21533=CARTESIAN_POINT('Ctrl Pts',(1.25722555095713,-0.388086240756494,
1.05871835910697));
#21534=CARTESIAN_POINT('Ctrl Pts',(1.27866649102984,-0.373586846396559,
1.03253285680459));
#21535=CARTESIAN_POINT('Ctrl Pts',(1.31521005565926,-0.33909093068465,0.985600426557816));
#21536=CARTESIAN_POINT('Ctrl Pts',(1.33211611256184,-0.317195968905306,
0.962485392528369));
#21537=CARTESIAN_POINT('Ctrl Pts',(1.36127834356734,-0.266264900654909,
0.920778333482565));
#21538=CARTESIAN_POINT('Ctrl Pts',(1.3735491215176,-0.237231147975234,0.902193646979983));
#21539=CARTESIAN_POINT('Ctrl Pts',(1.39550172959303,-0.166543350814306,
0.867957148219442));
#21540=CARTESIAN_POINT('Ctrl Pts',(1.40380622184538,-0.123401821157026,
0.854205272175555));
#21541=CARTESIAN_POINT('Ctrl Pts',(1.40825612658882,-0.0793800000000001,
0.846804978391753));
#21542=CARTESIAN_POINT('',(0.886256117232623,-0.07938,1.45861320581289));
#21543=CARTESIAN_POINT('Origin',(1.18440385848747,-0.07938,1.18440385848747));
#21544=CARTESIAN_POINT('',(1.45861320581289,-0.07938,0.886256117232624));
#21545=CARTESIAN_POINT('Ctrl Pts',(1.45861320581289,-0.0793800000000001,
0.886256117232623));
#21546=CARTESIAN_POINT('Ctrl Pts',(1.45630208793976,-0.101649918886749,
0.890059788636852));
#21547=CARTESIAN_POINT('Ctrl Pts',(1.45296717977858,-0.123823518623746,
0.895520212222107));
#21548=CARTESIAN_POINT('Ctrl Pts',(1.43904931717599,-0.192480977588836,
0.917859913453975));
#21549=CARTESIAN_POINT('Ctrl Pts',(1.4243271592157,-0.236152929235938,0.940896403863072));
#21550=CARTESIAN_POINT('Ctrl Pts',(1.39055359345152,-0.303141259068212,
0.990027513266106));
#21551=CARTESIAN_POINT('Ctrl Pts',(1.36743459453896,-0.335108247315849,
1.02199477007745));
#21552=CARTESIAN_POINT('Ctrl Pts',(1.32643091652006,-0.373243761060364,
1.07446535104584));
#21553=CARTESIAN_POINT('Ctrl Pts',(1.30441816675528,-0.387888272594439,
1.10126842659597));
#21554=CARTESIAN_POINT('Ctrl Pts',(1.25681160160691,-0.407041111792943,
1.15530234155453));
#21555=CARTESIAN_POINT('Ctrl Pts',(1.23119764287622,-0.411552957311693,
1.18251418313119));
#21556=CARTESIAN_POINT('Ctrl Pts',(1.18251418313119,-0.411552957311693,
1.23119764287622));
#21557=CARTESIAN_POINT('Ctrl Pts',(1.15530234155453,-0.407041111792943,
1.25681160160691));
#21558=CARTESIAN_POINT('Ctrl Pts',(1.10126842659597,-0.387888272594439,
1.30441816675528));
#21559=CARTESIAN_POINT('Ctrl Pts',(1.07446535104584,-0.373243761060364,
1.32643091652006));
#21560=CARTESIAN_POINT('Ctrl Pts',(1.02199477007745,-0.335108247315848,
1.36743459453896));
#21561=CARTESIAN_POINT('Ctrl Pts',(0.990027513266105,-0.303141259068211,
1.39055359345152));
#21562=CARTESIAN_POINT('Ctrl Pts',(0.940896403863071,-0.236152929235937,
1.42432715921571));
#21563=CARTESIAN_POINT('Ctrl Pts',(0.917859913453974,-0.192480977588835,
1.43904931717599));
#21564=CARTESIAN_POINT('Ctrl Pts',(0.895520212222106,-0.123823518623745,
1.45296717977858));
#21565=CARTESIAN_POINT('Ctrl Pts',(0.890059788636851,-0.101649918886749,
1.45630208793976));
#21566=CARTESIAN_POINT('Ctrl Pts',(0.886256117232622,-0.0793800000000001,
1.45861320581289));
#21567=CARTESIAN_POINT('Origin',(1.18440385848747,-0.07938,1.18440385848747));
#21568=CARTESIAN_POINT('Origin',(0.,-0.27783,0.));
#21569=CARTESIAN_POINT('',(0.404717578595295,-0.07938,1.65807299932179));
#21570=CARTESIAN_POINT('Origin',(0.,-0.07938,0.));
#21571=CARTESIAN_POINT('',(-0.404717578595296,-0.07938,1.65807299932179));
#21572=CARTESIAN_POINT('Ctrl Pts',(0.404717578595296,-0.0793800000000001,
1.65807299932179));
#21573=CARTESIAN_POINT('Ctrl Pts',(0.400393769631747,-0.101649918886749,
1.65912839404491));
#21574=CARTESIAN_POINT('Ctrl Pts',(0.394174530911058,-0.123823518623745,
1.66063136041479));
#21575=CARTESIAN_POINT('Ctrl Pts',(0.368536561654407,-0.192480977588835,
1.66658649961961));
#21576=CARTESIAN_POINT('Ctrl Pts',(0.341837165343982,-0.236152929235937,
1.67246562047521));
#21577=CARTESIAN_POINT('Ctrl Pts',(0.283214707341173,-0.303141259068211,
1.68332504372461));
#21578=CARTESIAN_POINT('Ctrl Pts',(0.244262842368623,-0.335108247315849,
1.68958170688653));
#21579=CARTESIAN_POINT('Ctrl Pts',(0.178166559972324,-0.373243761060364,
1.69769003172132));
#21580=CARTESIAN_POINT('Ctrl Pts',(0.143648558862931,-0.387888272594439,
1.70107730356824));
#21581=CARTESIAN_POINT('Ctrl Pts',(0.0717778861362652,-0.407041111792943,
1.70562212620408));
#21582=CARTESIAN_POINT('Ctrl Pts',(0.0344244045173309,-0.411552957311693,
1.706752));
#21583=CARTESIAN_POINT('Ctrl Pts',(-0.0344244045173315,-0.411552957311693,
1.706752));
#21584=CARTESIAN_POINT('Ctrl Pts',(-0.0717778861362658,-0.407041111792943,
1.70562212620408));
#21585=CARTESIAN_POINT('Ctrl Pts',(-0.143648558862932,-0.387888272594439,
1.70107730356824));
#21586=CARTESIAN_POINT('Ctrl Pts',(-0.178166559972325,-0.373243761060364,
1.69769003172132));
#21587=CARTESIAN_POINT('Ctrl Pts',(-0.244262842368624,-0.335108247315849,
1.68958170688653));
#21588=CARTESIAN_POINT('Ctrl Pts',(-0.283214707341173,-0.303141259068212,
1.68332504372461));
#21589=CARTESIAN_POINT('Ctrl Pts',(-0.341837165343982,-0.236152929235937,
1.67246562047521));
#21590=CARTESIAN_POINT('Ctrl Pts',(-0.368536561654408,-0.192480977588835,
1.66658649961961));
#21591=CARTESIAN_POINT('Ctrl Pts',(-0.394174530911059,-0.123823518623745,
1.66063136041479));
#21592=CARTESIAN_POINT('Ctrl Pts',(-0.400393769631748,-0.101649918886749,
1.65912839404491));
#21593=CARTESIAN_POINT('Ctrl Pts',(-0.404717578595297,-0.0793800000000001,
1.65807299932179));
#21594=CARTESIAN_POINT('',(-0.886256117232624,-0.07938,1.45861320581289));
#21595=CARTESIAN_POINT('Origin',(0.,-0.07938,0.));
#21596=CARTESIAN_POINT('',(-1.45861320581289,-0.07938,0.886256117232623));
#21597=CARTESIAN_POINT('Ctrl Pts',(-0.886256117232623,-0.0793800000000001,
1.45861320581289));
#21598=CARTESIAN_POINT('Ctrl Pts',(-0.890059788636852,-0.101649918886749,
1.45630208793976));
#21599=CARTESIAN_POINT('Ctrl Pts',(-0.895520212222106,-0.123823518623745,
1.45296717977858));
#21600=CARTESIAN_POINT('Ctrl Pts',(-0.917859913453974,-0.192480977588835,
1.43904931717599));
#21601=CARTESIAN_POINT('Ctrl Pts',(-0.940896403863071,-0.236152929235937,
1.4243271592157));
#21602=CARTESIAN_POINT('Ctrl Pts',(-0.990027513266105,-0.303141259068211,
1.39055359345152));
#21603=CARTESIAN_POINT('Ctrl Pts',(-1.02199477007745,-0.335108247315848,
1.36743459453896));
#21604=CARTESIAN_POINT('Ctrl Pts',(-1.07446535104584,-0.373243761060364,
1.32643091652006));
#21605=CARTESIAN_POINT('Ctrl Pts',(-1.10126842659597,-0.387888272594439,
1.30441816675528));
#21606=CARTESIAN_POINT('Ctrl Pts',(-1.15530234155453,-0.407041111792943,
1.25681160160691));
#21607=CARTESIAN_POINT('Ctrl Pts',(-1.18251418313119,-0.411552957311693,
1.23119764287622));
#21608=CARTESIAN_POINT('Ctrl Pts',(-1.23119764287622,-0.411552957311693,
1.18251418313119));
#21609=CARTESIAN_POINT('Ctrl Pts',(-1.25681160160691,-0.407041111792943,
1.15530234155453));
#21610=CARTESIAN_POINT('Ctrl Pts',(-1.30441816675528,-0.387888272594439,
1.10126842659597));
#21611=CARTESIAN_POINT('Ctrl Pts',(-1.32643091652006,-0.373243761060365,
1.07446535104584));
#21612=CARTESIAN_POINT('Ctrl Pts',(-1.36743459453896,-0.335108247315849,
1.02199477007745));
#21613=CARTESIAN_POINT('Ctrl Pts',(-1.39055359345152,-0.303141259068212,
0.990027513266106));
#21614=CARTESIAN_POINT('Ctrl Pts',(-1.4243271592157,-0.236152929235938,
0.940896403863071));
#21615=CARTESIAN_POINT('Ctrl Pts',(-1.43904931717599,-0.192480977588836,
0.917859913453974));
#21616=CARTESIAN_POINT('Ctrl Pts',(-1.45296717977858,-0.123823518623746,
0.895520212222106));
#21617=CARTESIAN_POINT('Ctrl Pts',(-1.45630208793976,-0.101649918886749,
0.890059788636852));
#21618=CARTESIAN_POINT('Ctrl Pts',(-1.45861320581289,-0.0793800000000001,
0.886256117232623));
#21619=CARTESIAN_POINT('',(-1.65807299932179,-0.07938,0.404717578595295));
#21620=CARTESIAN_POINT('Origin',(0.,-0.07938,0.));
#21621=CARTESIAN_POINT('',(-1.706752,-0.411552957311693,2.08591827245526E-16));
#21622=CARTESIAN_POINT('Ctrl Pts',(-1.65807299932179,-0.0793800000000001,
0.404717578595296));
#21623=CARTESIAN_POINT('Ctrl Pts',(-1.65912839404491,-0.101649918886749,
0.400393769631747));
#21624=CARTESIAN_POINT('Ctrl Pts',(-1.66063136041479,-0.123823518623745,
0.394174530911058));
#21625=CARTESIAN_POINT('Ctrl Pts',(-1.66658649961961,-0.192480977588835,
0.368536561654407));
#21626=CARTESIAN_POINT('Ctrl Pts',(-1.67246562047521,-0.236152929235937,
0.341837165343982));
#21627=CARTESIAN_POINT('Ctrl Pts',(-1.68332504372461,-0.303141259068211,
0.283214707341173));
#21628=CARTESIAN_POINT('Ctrl Pts',(-1.68958170688653,-0.335108247315848,
0.244262842368623));
#21629=CARTESIAN_POINT('Ctrl Pts',(-1.69769003172132,-0.373243761060364,
0.178166559972324));
#21630=CARTESIAN_POINT('Ctrl Pts',(-1.70107730356824,-0.387888272594439,
0.143648558862931));
#21631=CARTESIAN_POINT('Ctrl Pts',(-1.70562212620408,-0.407041111792943,
0.0717778861362656));
#21632=CARTESIAN_POINT('Ctrl Pts',(-1.706752,-0.411552957311693,0.0344244045173313));
#21633=CARTESIAN_POINT('Ctrl Pts',(-1.706752,-0.411552957311693,2.08166817117217E-16));
#21634=CARTESIAN_POINT('',(-1.706752,-0.47628,2.09016837373834E-16));
#21635=CARTESIAN_POINT('',(-1.706752,-0.27783,2.09016837373834E-16));
#21636=CARTESIAN_POINT('Origin',(0.,-0.47628,0.));
#21637=CARTESIAN_POINT('',(-1.65807299932179,-0.07938,-0.404717578595296));
#21638=CARTESIAN_POINT('Ctrl Pts',(-1.706752,-0.411552957311693,2.0122792321331E-16));
#21639=CARTESIAN_POINT('Ctrl Pts',(-1.706752,-0.411552957311693,-0.0344244045173309));
#21640=CARTESIAN_POINT('Ctrl Pts',(-1.70562212620408,-0.407041111792943,
-0.0717778861362652));
#21641=CARTESIAN_POINT('Ctrl Pts',(-1.70107730356824,-0.387888272594439,
-0.143648558862931));
#21642=CARTESIAN_POINT('Ctrl Pts',(-1.69769003172132,-0.373243761060365,
-0.178166559972324));
#21643=CARTESIAN_POINT('Ctrl Pts',(-1.68958170688653,-0.335108247315849,
-0.244262842368623));
#21644=CARTESIAN_POINT('Ctrl Pts',(-1.68332504372461,-0.303141259068212,
-0.283214707341173));
#21645=CARTESIAN_POINT('Ctrl Pts',(-1.67246562047521,-0.236152929235938,
-0.341837165343982));
#21646=CARTESIAN_POINT('Ctrl Pts',(-1.66658649961961,-0.192480977588836,
-0.368536561654407));
#21647=CARTESIAN_POINT('Ctrl Pts',(-1.66063136041479,-0.123823518623745,
-0.394174530911059));
#21648=CARTESIAN_POINT('Ctrl Pts',(-1.65912839404491,-0.101649918886749,
-0.400393769631748));
#21649=CARTESIAN_POINT('Ctrl Pts',(-1.65807299932179,-0.0793800000000001,
-0.404717578595296));
#21650=CARTESIAN_POINT('',(-1.45861320581289,-0.07938,-0.886256117232623));
#21651=CARTESIAN_POINT('Origin',(0.,-0.07938,0.));
#21652=CARTESIAN_POINT('',(-0.886256117232623,-0.07938,-1.45861320581289));
#21653=CARTESIAN_POINT('Ctrl Pts',(-1.45861320581289,-0.0793800000000001,
-0.886256117232623));
#21654=CARTESIAN_POINT('Ctrl Pts',(-1.45630208793976,-0.101649918886749,
-0.890059788636852));
#21655=CARTESIAN_POINT('Ctrl Pts',(-1.45296717977858,-0.123823518623745,
-0.895520212222106));
#21656=CARTESIAN_POINT('Ctrl Pts',(-1.43904931717599,-0.192480977588835,
-0.917859913453974));
#21657=CARTESIAN_POINT('Ctrl Pts',(-1.4243271592157,-0.236152929235937,
-0.940896403863072));
#21658=CARTESIAN_POINT('Ctrl Pts',(-1.39055359345152,-0.303141259068212,
-0.990027513266106));
#21659=CARTESIAN_POINT('Ctrl Pts',(-1.36743459453896,-0.335108247315849,
-1.02199477007745));
#21660=CARTESIAN_POINT('Ctrl Pts',(-1.32643091652006,-0.373243761060364,
-1.07446535104584));
#21661=CARTESIAN_POINT('Ctrl Pts',(-1.30441816675528,-0.387888272594439,
-1.10126842659597));
#21662=CARTESIAN_POINT('Ctrl Pts',(-1.25681160160691,-0.407041111792943,
-1.15530234155453));
#21663=CARTESIAN_POINT('Ctrl Pts',(-1.23119764287622,-0.411552957311693,
-1.18251418313119));
#21664=CARTESIAN_POINT('Ctrl Pts',(-1.18251418313119,-0.411552957311693,
-1.23119764287622));
#21665=CARTESIAN_POINT('Ctrl Pts',(-1.15530234155453,-0.407041111792943,
-1.25681160160691));
#21666=CARTESIAN_POINT('Ctrl Pts',(-1.10126842659597,-0.387888272594439,
-1.30441816675528));
#21667=CARTESIAN_POINT('Ctrl Pts',(-1.07446535104584,-0.373243761060364,
-1.32643091652006));
#21668=CARTESIAN_POINT('Ctrl Pts',(-1.02199477007745,-0.335108247315848,
-1.36743459453896));
#21669=CARTESIAN_POINT('Ctrl Pts',(-0.990027513266105,-0.303141259068211,
-1.39055359345152));
#21670=CARTESIAN_POINT('Ctrl Pts',(-0.940896403863071,-0.236152929235936,
-1.42432715921571));
#21671=CARTESIAN_POINT('Ctrl Pts',(-0.917859913453974,-0.192480977588835,
-1.43904931717599));
#21672=CARTESIAN_POINT('Ctrl Pts',(-0.895520212222106,-0.123823518623745,
-1.45296717977858));
#21673=CARTESIAN_POINT('Ctrl Pts',(-0.890059788636851,-0.101649918886749,
-1.45630208793976));
#21674=CARTESIAN_POINT('Ctrl Pts',(-0.886256117232623,-0.0793800000000001,
-1.45861320581289));
#21675=CARTESIAN_POINT('',(-0.404717578595295,-0.07938,-1.65807299932179));
#21676=CARTESIAN_POINT('Origin',(0.,-0.07938,0.));
#21677=CARTESIAN_POINT('',(0.404717578595296,-0.07938,-1.65807299932179));
#21678=CARTESIAN_POINT('Ctrl Pts',(-0.404717578595296,-0.0793800000000001,
-1.65807299932179));
#21679=CARTESIAN_POINT('Ctrl Pts',(-0.400393769631747,-0.101649918886749,
-1.65912839404491));
#21680=CARTESIAN_POINT('Ctrl Pts',(-0.394174530911058,-0.123823518623746,
-1.66063136041479));
#21681=CARTESIAN_POINT('Ctrl Pts',(-0.368536561654407,-0.192480977588836,
-1.66658649961961));
#21682=CARTESIAN_POINT('Ctrl Pts',(-0.341837165343982,-0.236152929235938,
-1.67246562047521));
#21683=CARTESIAN_POINT('Ctrl Pts',(-0.283214707341173,-0.303141259068212,
-1.68332504372461));
#21684=CARTESIAN_POINT('Ctrl Pts',(-0.244262842368623,-0.335108247315849,
-1.68958170688653));
#21685=CARTESIAN_POINT('Ctrl Pts',(-0.178166559972324,-0.373243761060364,
-1.69769003172132));
#21686=CARTESIAN_POINT('Ctrl Pts',(-0.143648558862931,-0.387888272594439,
-1.70107730356824));
#21687=CARTESIAN_POINT('Ctrl Pts',(-0.0717778861362653,-0.407041111792943,
-1.70562212620408));
#21688=CARTESIAN_POINT('Ctrl Pts',(-0.034424404517331,-0.411552957311693,
-1.706752));
#21689=CARTESIAN_POINT('Ctrl Pts',(0.0344244045173312,-0.411552957311693,
-1.706752));
#21690=CARTESIAN_POINT('Ctrl Pts',(0.0717778861362655,-0.407041111792943,
-1.70562212620408));
#21691=CARTESIAN_POINT('Ctrl Pts',(0.143648558862931,-0.387888272594439,
-1.70107730356824));
#21692=CARTESIAN_POINT('Ctrl Pts',(0.178166559972324,-0.373243761060364,
-1.69769003172132));
#21693=CARTESIAN_POINT('Ctrl Pts',(0.244262842368623,-0.335108247315849,
-1.68958170688653));
#21694=CARTESIAN_POINT('Ctrl Pts',(0.283214707341173,-0.303141259068212,
-1.68332504372461));
#21695=CARTESIAN_POINT('Ctrl Pts',(0.341837165343982,-0.236152929235937,
-1.67246562047521));
#21696=CARTESIAN_POINT('Ctrl Pts',(0.368536561654407,-0.192480977588835,
-1.66658649961961));
#21697=CARTESIAN_POINT('Ctrl Pts',(0.394174530911059,-0.123823518623745,
-1.66063136041479));
#21698=CARTESIAN_POINT('Ctrl Pts',(0.400393769631748,-0.101649918886749,
-1.65912839404491));
#21699=CARTESIAN_POINT('Ctrl Pts',(0.404717578595296,-0.0793800000000001,
-1.65807299932179));
#21700=CARTESIAN_POINT('',(0.886256117232623,-0.07938,-1.45861320581289));
#21701=CARTESIAN_POINT('Origin',(0.,-0.07938,0.));
#21702=CARTESIAN_POINT('',(1.45861320581289,-0.07938,-0.886256117232623));
#21703=CARTESIAN_POINT('Ctrl Pts',(0.886256117232623,-0.0793800000000001,
-1.45861320581289));
#21704=CARTESIAN_POINT('Ctrl Pts',(0.890059788636852,-0.101649918886749,
-1.45630208793976));
#21705=CARTESIAN_POINT('Ctrl Pts',(0.895520212222106,-0.123823518623745,
-1.45296717977858));
#21706=CARTESIAN_POINT('Ctrl Pts',(0.917859913453974,-0.192480977588835,
-1.43904931717599));
#21707=CARTESIAN_POINT('Ctrl Pts',(0.940896403863072,-0.236152929235937,
-1.4243271592157));
#21708=CARTESIAN_POINT('Ctrl Pts',(0.990027513266106,-0.303141259068211,
-1.39055359345152));
#21709=CARTESIAN_POINT('Ctrl Pts',(1.02199477007745,-0.335108247315849,
-1.36743459453896));
#21710=CARTESIAN_POINT('Ctrl Pts',(1.07446535104584,-0.373243761060364,
-1.32643091652006));
#21711=CARTESIAN_POINT('Ctrl Pts',(1.10126842659597,-0.387888272594439,
-1.30441816675528));
#21712=CARTESIAN_POINT('Ctrl Pts',(1.15530234155453,-0.407041111792943,
-1.25681160160691));
#21713=CARTESIAN_POINT('Ctrl Pts',(1.18251418313119,-0.411552957311693,
-1.23119764287622));
#21714=CARTESIAN_POINT('Ctrl Pts',(1.23119764287622,-0.411552957311693,
-1.18251418313119));
#21715=CARTESIAN_POINT('Ctrl Pts',(1.25681160160691,-0.407041111792943,
-1.15530234155453));
#21716=CARTESIAN_POINT('Ctrl Pts',(1.30441816675528,-0.387888272594439,
-1.10126842659597));
#21717=CARTESIAN_POINT('Ctrl Pts',(1.32643091652006,-0.373243761060364,
-1.07446535104584));
#21718=CARTESIAN_POINT('Ctrl Pts',(1.36743459453896,-0.335108247315849,
-1.02199477007745));
#21719=CARTESIAN_POINT('Ctrl Pts',(1.39055359345152,-0.303141259068212,
-0.990027513266105));
#21720=CARTESIAN_POINT('Ctrl Pts',(1.4243271592157,-0.236152929235937,-0.940896403863071));
#21721=CARTESIAN_POINT('Ctrl Pts',(1.43904931717599,-0.192480977588835,
-0.917859913453974));
#21722=CARTESIAN_POINT('Ctrl Pts',(1.45296717977858,-0.123823518623745,
-0.895520212222106));
#21723=CARTESIAN_POINT('Ctrl Pts',(1.45630208793976,-0.101649918886749,
-0.890059788636852));
#21724=CARTESIAN_POINT('Ctrl Pts',(1.45861320581289,-0.0793800000000001,
-0.886256117232623));
#21725=CARTESIAN_POINT('',(1.65807299932179,-0.07938,-0.404717578595296));
#21726=CARTESIAN_POINT('Origin',(0.,-0.07938,0.));
#21727=CARTESIAN_POINT('',(1.65807299932179,-0.07938,0.404717578595296));
#21728=CARTESIAN_POINT('Ctrl Pts',(1.65807299932179,-0.0793800000000001,
-0.404717578595296));
#21729=CARTESIAN_POINT('Ctrl Pts',(1.65912839404491,-0.101649918886749,
-0.400393769631747));
#21730=CARTESIAN_POINT('Ctrl Pts',(1.66063136041479,-0.123823518623745,
-0.394174530911058));
#21731=CARTESIAN_POINT('Ctrl Pts',(1.66658649961961,-0.192480977588835,
-0.368536561654407));
#21732=CARTESIAN_POINT('Ctrl Pts',(1.67246562047521,-0.236152929235937,
-0.341837165343982));
#21733=CARTESIAN_POINT('Ctrl Pts',(1.68332504372461,-0.303141259068212,
-0.283214707341173));
#21734=CARTESIAN_POINT('Ctrl Pts',(1.68958170688653,-0.335108247315849,
-0.244262842368623));
#21735=CARTESIAN_POINT('Ctrl Pts',(1.69769003172132,-0.373243761060364,
-0.178166559972324));
#21736=CARTESIAN_POINT('Ctrl Pts',(1.70107730356824,-0.387888272594439,
-0.143648558862931));
#21737=CARTESIAN_POINT('Ctrl Pts',(1.70562212620408,-0.407041111792943,
-0.0717778861362655));
#21738=CARTESIAN_POINT('Ctrl Pts',(1.706752,-0.411552957311693,-0.0344244045173312));
#21739=CARTESIAN_POINT('Ctrl Pts',(1.706752,-0.411552957311693,0.0344244045173312));
#21740=CARTESIAN_POINT('Ctrl Pts',(1.70562212620408,-0.407041111792943,
0.0717778861362655));
#21741=CARTESIAN_POINT('Ctrl Pts',(1.70107730356824,-0.387888272594439,
0.143648558862931));
#21742=CARTESIAN_POINT('Ctrl Pts',(1.69769003172132,-0.373243761060364,
0.178166559972324));
#21743=CARTESIAN_POINT('Ctrl Pts',(1.68958170688653,-0.335108247315849,
0.244262842368623));
#21744=CARTESIAN_POINT('Ctrl Pts',(1.68332504372461,-0.303141259068212,
0.283214707341173));
#21745=CARTESIAN_POINT('Ctrl Pts',(1.67246562047521,-0.236152929235937,
0.341837165343982));
#21746=CARTESIAN_POINT('Ctrl Pts',(1.66658649961961,-0.192480977588835,
0.368536561654407));
#21747=CARTESIAN_POINT('Ctrl Pts',(1.66063136041479,-0.123823518623745,
0.394174530911058));
#21748=CARTESIAN_POINT('Ctrl Pts',(1.65912839404491,-0.101649918886749,
0.400393769631747));
#21749=CARTESIAN_POINT('Ctrl Pts',(1.65807299932179,-0.0793800000000001,
0.404717578595296));
#21750=CARTESIAN_POINT('Origin',(0.,-0.07938,0.));
#21751=CARTESIAN_POINT('Origin',(0.,-0.07938,0.));
#21752=CARTESIAN_POINT('',(0.397005914195118,-0.07938,1.59456899932179));
#21753=CARTESIAN_POINT('Origin',(0.,-0.07938,0.));
#21754=CARTESIAN_POINT('Origin',(-3.33066907387547E-16,-0.07938,1.675));
#21755=CARTESIAN_POINT('Origin',(-3.33066907387547E-16,0.,1.675));
#21756=CARTESIAN_POINT('',(-0.397005914195118,-0.07938,1.59456899932179));
#21757=CARTESIAN_POINT('Ctrl Pts',(-0.397005914195119,-0.0793800000000001,
1.59456899932179));
#21758=CARTESIAN_POINT('Ctrl Pts',(-0.3886265584581,-0.123401821157026,
1.59665523941937));
#21759=CARTESIAN_POINT('Ctrl Pts',(-0.373030350867485,-0.166543350814306,
1.60050712143809));
#21760=CARTESIAN_POINT('Ctrl Pts',(-0.333298652394954,-0.237231147975234,
1.60919314384089));
#21761=CARTESIAN_POINT('Ctrl Pts',(-0.311480544243687,-0.266264900654909,
1.61365775139403));
#21762=CARTESIAN_POINT('Ctrl Pts',(-0.261368388670537,-0.317195968905306,
1.62252828437015));
#21763=CARTESIAN_POINT('Ctrl Pts',(-0.233069203882014,-0.33909093068465,
1.62691869420078));
#21764=CARTESIAN_POINT('Ctrl Pts',(-0.174042761838764,-0.373586846396559,
1.63426473152765));
#21765=CARTESIAN_POINT('Ctrl Pts',(-0.14036578147155,-0.388086240756494,
1.63761964365402));
#21766=CARTESIAN_POINT('Ctrl Pts',(-0.0701778381840615,-0.407068917407805,
1.64212536811722));
#21767=CARTESIAN_POINT('Ctrl Pts',(-0.0336652739555918,-0.411552957311693,
1.643248));
#21768=CARTESIAN_POINT('Ctrl Pts',(0.0336652739555913,-0.411552957311693,
1.643248));
#21769=CARTESIAN_POINT('Ctrl Pts',(0.070177838184061,-0.407068917407805,
1.64212536811722));
#21770=CARTESIAN_POINT('Ctrl Pts',(0.140365781471549,-0.388086240756494,
1.63761964365402));
#21771=CARTESIAN_POINT('Ctrl Pts',(0.174042761838763,-0.373586846396559,
1.63426473152765));
#21772=CARTESIAN_POINT('Ctrl Pts',(0.233069203882014,-0.33909093068465,
1.62691869420078));
#21773=CARTESIAN_POINT('Ctrl Pts',(0.261368388670536,-0.317195968905306,
1.62252828437015));
#21774=CARTESIAN_POINT('Ctrl Pts',(0.311480544243686,-0.266264900654908,
1.61365775139403));
#21775=CARTESIAN_POINT('Ctrl Pts',(0.333298652394954,-0.237231147975234,
1.60919314384089));
#21776=CARTESIAN_POINT('Ctrl Pts',(0.373030350867484,-0.166543350814306,
1.60050712143809));
#21777=CARTESIAN_POINT('Ctrl Pts',(0.388626558458099,-0.123401821157026,
1.59665523941937));
#21778=CARTESIAN_POINT('Ctrl Pts',(0.397005914195118,-0.07938,1.59456899932179));
#21779=CARTESIAN_POINT('Origin',(-3.33066907387547E-16,-0.07938,1.675));
#21780=CARTESIAN_POINT('Origin',(0.,-0.07938,0.));
#21781=CARTESIAN_POINT('',(-0.846804978391754,-0.07938,1.40825612658882));
#21782=CARTESIAN_POINT('Origin',(0.,-0.07938,0.));
#21783=CARTESIAN_POINT('Origin',(-1.18440385848747,-0.07938,1.18440385848747));
#21784=CARTESIAN_POINT('Origin',(-1.18440385848747,0.,1.18440385848747));
#21785=CARTESIAN_POINT('',(-1.40825612658882,-0.07938,0.846804978391753));
#21786=CARTESIAN_POINT('Ctrl Pts',(-1.40825612658882,-0.0793800000000001,
0.846804978391753));
#21787=CARTESIAN_POINT('Ctrl Pts',(-1.40380622184538,-0.123401821157026,
0.854205272175555));
#21788=CARTESIAN_POINT('Ctrl Pts',(-1.39550172959303,-0.166543350814306,
0.867957148219442));
#21789=CARTESIAN_POINT('Ctrl Pts',(-1.3735491215176,-0.237231147975235,
0.902193646979983));
#21790=CARTESIAN_POINT('Ctrl Pts',(-1.36127834356734,-0.266264900654909,
0.920778333482565));
#21791=CARTESIAN_POINT('Ctrl Pts',(-1.33211611256184,-0.317195968905306,
0.962485392528369));
#21792=CARTESIAN_POINT('Ctrl Pts',(-1.31521005565926,-0.339090930684651,
0.985600426557816));
#21793=CARTESIAN_POINT('Ctrl Pts',(-1.27866649102984,-0.373586846396559,
1.03253285680459));
#21794=CARTESIAN_POINT('Ctrl Pts',(-1.25722555095714,-0.388086240756494,
1.05871835910697));
#21795=CARTESIAN_POINT('Ctrl Pts',(-1.2107812086231,-0.407068917407805,
1.11153475808518));
#21796=CARTESIAN_POINT('Ctrl Pts',(-1.18575674747573,-0.411552957311693,
1.13814686046673));
#21797=CARTESIAN_POINT('Ctrl Pts',(-1.13814686046673,-0.411552957311693,
1.18575674747573));
#21798=CARTESIAN_POINT('Ctrl Pts',(-1.11153475808518,-0.407068917407805,
1.2107812086231));
#21799=CARTESIAN_POINT('Ctrl Pts',(-1.05871835910697,-0.388086240756494,
1.25722555095714));
#21800=CARTESIAN_POINT('Ctrl Pts',(-1.03253285680459,-0.373586846396559,
1.27866649102984));
#21801=CARTESIAN_POINT('Ctrl Pts',(-0.985600426557816,-0.33909093068465,
1.31521005565926));
#21802=CARTESIAN_POINT('Ctrl Pts',(-0.962485392528369,-0.317195968905306,
1.33211611256184));
#21803=CARTESIAN_POINT('Ctrl Pts',(-0.920778333482565,-0.266264900654908,
1.36127834356734));
#21804=CARTESIAN_POINT('Ctrl Pts',(-0.902193646979983,-0.237231147975234,
1.3735491215176));
#21805=CARTESIAN_POINT('Ctrl Pts',(-0.867957148219442,-0.166543350814306,
1.39550172959303));
#21806=CARTESIAN_POINT('Ctrl Pts',(-0.854205272175555,-0.123401821157026,
1.40380622184538));
#21807=CARTESIAN_POINT('Ctrl Pts',(-0.846804978391753,-0.0793800000000001,
1.40825612658882));
#21808=CARTESIAN_POINT('Origin',(-1.18440385848747,-0.07938,1.18440385848747));
#21809=CARTESIAN_POINT('Origin',(0.,-0.07938,0.));
#21810=CARTESIAN_POINT('',(-1.59456899932179,-0.07938,0.397005914195118));
#21811=CARTESIAN_POINT('Origin',(0.,-0.07938,0.));
#21812=CARTESIAN_POINT('Origin',(-1.675,-0.07938,-2.22044604925031E-16));
#21813=CARTESIAN_POINT('Origin',(-1.675,0.,-2.22044604925031E-16));
#21814=CARTESIAN_POINT('',(-1.59456899932179,-0.07938,-0.397005914195118));
#21815=CARTESIAN_POINT('',(-1.643248,-0.411552957311693,3.47540551556327E-18));
#21816=CARTESIAN_POINT('Ctrl Pts',(-1.59456899932179,-0.0793800000000001,
-0.397005914195119));
#21817=CARTESIAN_POINT('Ctrl Pts',(-1.59665523941937,-0.123401821157026,
-0.388626558458099));
#21818=CARTESIAN_POINT('Ctrl Pts',(-1.60050712143809,-0.166543350814306,
-0.373030350867485));
#21819=CARTESIAN_POINT('Ctrl Pts',(-1.60919314384089,-0.237231147975234,
-0.333298652394954));
#21820=CARTESIAN_POINT('Ctrl Pts',(-1.61365775139403,-0.266264900654909,
-0.311480544243686));
#21821=CARTESIAN_POINT('Ctrl Pts',(-1.62252828437015,-0.317195968905306,
-0.261368388670537));
#21822=CARTESIAN_POINT('Ctrl Pts',(-1.62691869420078,-0.33909093068465,
-0.233069203882014));
#21823=CARTESIAN_POINT('Ctrl Pts',(-1.63426473152765,-0.373586846396559,
-0.174042761838764));
#21824=CARTESIAN_POINT('Ctrl Pts',(-1.63761964365402,-0.388086240756494,
-0.140365781471549));
#21825=CARTESIAN_POINT('Ctrl Pts',(-1.64212536811722,-0.407068917407805,
-0.0701778381840614));
#21826=CARTESIAN_POINT('Ctrl Pts',(-1.643248,-0.411552957311693,-0.0336652739555917));
#21827=CARTESIAN_POINT('Ctrl Pts',(-1.643248,-0.411552957311693,-2.0122792321331E-16));
#21828=CARTESIAN_POINT('Origin',(-1.675,-0.07938,-2.22044604925031E-16));
#21829=CARTESIAN_POINT('Ctrl Pts',(-1.643248,-0.411552957311693,-1.94289029309402E-16));
#21830=CARTESIAN_POINT('Ctrl Pts',(-1.643248,-0.411552957311693,0.0336652739555913));
#21831=CARTESIAN_POINT('Ctrl Pts',(-1.64212536811722,-0.407068917407805,
0.0701778381840609));
#21832=CARTESIAN_POINT('Ctrl Pts',(-1.63761964365402,-0.388086240756494,
0.140365781471549));
#21833=CARTESIAN_POINT('Ctrl Pts',(-1.63426473152765,-0.373586846396559,
0.174042761838763));
#21834=CARTESIAN_POINT('Ctrl Pts',(-1.62691869420078,-0.33909093068465,
0.233069203882014));
#21835=CARTESIAN_POINT('Ctrl Pts',(-1.62252828437015,-0.317195968905306,
0.261368388670536));
#21836=CARTESIAN_POINT('Ctrl Pts',(-1.61365775139403,-0.266264900654909,
0.311480544243686));
#21837=CARTESIAN_POINT('Ctrl Pts',(-1.60919314384089,-0.237231147975235,
0.333298652394954));
#21838=CARTESIAN_POINT('Ctrl Pts',(-1.60050712143809,-0.166543350814306,
0.373030350867484));
#21839=CARTESIAN_POINT('Ctrl Pts',(-1.59665523941937,-0.123401821157026,
0.388626558458099));
#21840=CARTESIAN_POINT('Ctrl Pts',(-1.59456899932179,-0.0793800000000001,
0.397005914195118));
#21841=CARTESIAN_POINT('Origin',(0.,-0.07938,0.));
#21842=CARTESIAN_POINT('',(-1.40825612658882,-0.07938,-0.846804978391753));
#21843=CARTESIAN_POINT('Origin',(0.,-0.07938,0.));
#21844=CARTESIAN_POINT('Origin',(-1.18440385848747,-0.07938,-1.18440385848747));
#21845=CARTESIAN_POINT('Origin',(-1.18440385848747,0.,-1.18440385848747));
#21846=CARTESIAN_POINT('',(-0.846804978391753,-0.07938,-1.40825612658882));
#21847=CARTESIAN_POINT('Ctrl Pts',(-0.846804978391753,-0.0793800000000001,
-1.40825612658882));
#21848=CARTESIAN_POINT('Ctrl Pts',(-0.854205272175555,-0.123401821157026,
-1.40380622184538));
#21849=CARTESIAN_POINT('Ctrl Pts',(-0.867957148219442,-0.166543350814306,
-1.39550172959303));
#21850=CARTESIAN_POINT('Ctrl Pts',(-0.902193646979982,-0.237231147975234,
-1.3735491215176));
#21851=CARTESIAN_POINT('Ctrl Pts',(-0.920778333482564,-0.266264900654908,
-1.36127834356734));
#21852=CARTESIAN_POINT('Ctrl Pts',(-0.962485392528368,-0.317195968905306,
-1.33211611256184));
#21853=CARTESIAN_POINT('Ctrl Pts',(-0.985600426557816,-0.33909093068465,
-1.31521005565926));
#21854=CARTESIAN_POINT('Ctrl Pts',(-1.03253285680459,-0.373586846396559,
-1.27866649102984));
#21855=CARTESIAN_POINT('Ctrl Pts',(-1.05871835910697,-0.388086240756494,
-1.25722555095714));
#21856=CARTESIAN_POINT('Ctrl Pts',(-1.11153475808518,-0.407068917407805,
-1.2107812086231));
#21857=CARTESIAN_POINT('Ctrl Pts',(-1.13814686046673,-0.411552957311693,
-1.18575674747573));
#21858=CARTESIAN_POINT('Ctrl Pts',(-1.18575674747573,-0.411552957311693,
-1.13814686046673));
#21859=CARTESIAN_POINT('Ctrl Pts',(-1.2107812086231,-0.407068917407805,
-1.11153475808518));
#21860=CARTESIAN_POINT('Ctrl Pts',(-1.25722555095714,-0.388086240756494,
-1.05871835910697));
#21861=CARTESIAN_POINT('Ctrl Pts',(-1.27866649102984,-0.373586846396559,
-1.03253285680459));
#21862=CARTESIAN_POINT('Ctrl Pts',(-1.31521005565926,-0.33909093068465,
-0.985600426557816));
#21863=CARTESIAN_POINT('Ctrl Pts',(-1.33211611256184,-0.317195968905306,
-0.962485392528369));
#21864=CARTESIAN_POINT('Ctrl Pts',(-1.36127834356734,-0.266264900654909,
-0.920778333482565));
#21865=CARTESIAN_POINT('Ctrl Pts',(-1.3735491215176,-0.237231147975234,
-0.902193646979983));
#21866=CARTESIAN_POINT('Ctrl Pts',(-1.39550172959303,-0.166543350814306,
-0.867957148219442));
#21867=CARTESIAN_POINT('Ctrl Pts',(-1.40380622184538,-0.123401821157026,
-0.854205272175555));
#21868=CARTESIAN_POINT('Ctrl Pts',(-1.40825612658882,-0.07938,-0.846804978391753));
#21869=CARTESIAN_POINT('Origin',(-1.18440385848747,-0.07938,-1.18440385848747));
#21870=CARTESIAN_POINT('Origin',(0.,-0.07938,0.));
#21871=CARTESIAN_POINT('',(-0.397005914195118,-0.07938,-1.59456899932179));
#21872=CARTESIAN_POINT('Origin',(0.,-0.07938,0.));
#21873=CARTESIAN_POINT('Origin',(1.11022302462516E-16,-0.07938,-1.675));
#21874=CARTESIAN_POINT('Origin',(1.11022302462516E-16,0.,-1.675));
#21875=CARTESIAN_POINT('',(0.397005914195118,-0.07938,-1.59456899932179));
#21876=CARTESIAN_POINT('Ctrl Pts',(0.397005914195119,-0.0793800000000001,
-1.59456899932179));
#21877=CARTESIAN_POINT('Ctrl Pts',(0.388626558458099,-0.123401821157026,
-1.59665523941937));
#21878=CARTESIAN_POINT('Ctrl Pts',(0.373030350867485,-0.166543350814306,
-1.60050712143809));
#21879=CARTESIAN_POINT('Ctrl Pts',(0.333298652394954,-0.237231147975234,
-1.60919314384089));
#21880=CARTESIAN_POINT('Ctrl Pts',(0.311480544243686,-0.266264900654909,
-1.61365775139403));
#21881=CARTESIAN_POINT('Ctrl Pts',(0.261368388670537,-0.317195968905306,
-1.62252828437015));
#21882=CARTESIAN_POINT('Ctrl Pts',(0.233069203882014,-0.33909093068465,
-1.62691869420078));
#21883=CARTESIAN_POINT('Ctrl Pts',(0.174042761838763,-0.373586846396559,
-1.63426473152765));
#21884=CARTESIAN_POINT('Ctrl Pts',(0.140365781471549,-0.388086240756494,
-1.63761964365402));
#21885=CARTESIAN_POINT('Ctrl Pts',(0.0701778381840612,-0.407068917407805,
-1.64212536811722));
#21886=CARTESIAN_POINT('Ctrl Pts',(0.0336652739555916,-0.411552957311693,
-1.643248));
#21887=CARTESIAN_POINT('Ctrl Pts',(-0.0336652739555915,-0.411552957311693,
-1.643248));
#21888=CARTESIAN_POINT('Ctrl Pts',(-0.0701778381840612,-0.407068917407805,
-1.64212536811722));
#21889=CARTESIAN_POINT('Ctrl Pts',(-0.140365781471549,-0.388086240756494,
-1.63761964365402));
#21890=CARTESIAN_POINT('Ctrl Pts',(-0.174042761838764,-0.373586846396559,
-1.63426473152765));
#21891=CARTESIAN_POINT('Ctrl Pts',(-0.233069203882014,-0.33909093068465,
-1.62691869420078));
#21892=CARTESIAN_POINT('Ctrl Pts',(-0.261368388670536,-0.317195968905306,
-1.62252828437015));
#21893=CARTESIAN_POINT('Ctrl Pts',(-0.311480544243686,-0.266264900654908,
-1.61365775139403));
#21894=CARTESIAN_POINT('Ctrl Pts',(-0.333298652394954,-0.237231147975234,
-1.60919314384089));
#21895=CARTESIAN_POINT('Ctrl Pts',(-0.373030350867485,-0.166543350814306,
-1.60050712143809));
#21896=CARTESIAN_POINT('Ctrl Pts',(-0.388626558458099,-0.123401821157026,
-1.59665523941937));
#21897=CARTESIAN_POINT('Ctrl Pts',(-0.397005914195118,-0.07938,-1.59456899932179));
#21898=CARTESIAN_POINT('Origin',(1.11022302462516E-16,-0.07938,-1.675));
#21899=CARTESIAN_POINT('Origin',(0.,-0.07938,0.));
#21900=CARTESIAN_POINT('',(0.846804978391753,-0.07938,-1.40825612658882));
#21901=CARTESIAN_POINT('Origin',(0.,-0.07938,0.));
#21902=CARTESIAN_POINT('Origin',(1.18440385848747,-0.07938,-1.18440385848747));
#21903=CARTESIAN_POINT('Origin',(1.18440385848747,0.,-1.18440385848747));
#21904=CARTESIAN_POINT('',(1.40825612658882,-0.07938,-0.846804978391753));
#21905=CARTESIAN_POINT('Ctrl Pts',(1.40825612658882,-0.0793800000000001,
-0.846804978391753));
#21906=CARTESIAN_POINT('Ctrl Pts',(1.40380622184538,-0.123401821157026,
-0.854205272175555));
#21907=CARTESIAN_POINT('Ctrl Pts',(1.39550172959303,-0.166543350814306,
-0.867957148219442));
#21908=CARTESIAN_POINT('Ctrl Pts',(1.3735491215176,-0.237231147975234,-0.902193646979983));
#21909=CARTESIAN_POINT('Ctrl Pts',(1.36127834356734,-0.266264900654908,
-0.920778333482565));
#21910=CARTESIAN_POINT('Ctrl Pts',(1.33211611256184,-0.317195968905306,
-0.962485392528369));
#21911=CARTESIAN_POINT('Ctrl Pts',(1.31521005565926,-0.33909093068465,-0.985600426557816));
#21912=CARTESIAN_POINT('Ctrl Pts',(1.27866649102984,-0.373586846396559,
-1.03253285680459));
#21913=CARTESIAN_POINT('Ctrl Pts',(1.25722555095714,-0.388086240756494,
-1.05871835910697));
#21914=CARTESIAN_POINT('Ctrl Pts',(1.2107812086231,-0.407068917407805,-1.11153475808518));
#21915=CARTESIAN_POINT('Ctrl Pts',(1.18575674747573,-0.411552957311693,
-1.13814686046673));
#21916=CARTESIAN_POINT('Ctrl Pts',(1.13814686046673,-0.411552957311693,
-1.18575674747573));
#21917=CARTESIAN_POINT('Ctrl Pts',(1.11153475808518,-0.407068917407805,
-1.2107812086231));
#21918=CARTESIAN_POINT('Ctrl Pts',(1.05871835910697,-0.388086240756494,
-1.25722555095714));
#21919=CARTESIAN_POINT('Ctrl Pts',(1.03253285680459,-0.373586846396559,
-1.27866649102984));
#21920=CARTESIAN_POINT('Ctrl Pts',(0.985600426557816,-0.33909093068465,
-1.31521005565926));
#21921=CARTESIAN_POINT('Ctrl Pts',(0.962485392528369,-0.317195968905306,
-1.33211611256184));
#21922=CARTESIAN_POINT('Ctrl Pts',(0.920778333482565,-0.266264900654909,
-1.36127834356734));
#21923=CARTESIAN_POINT('Ctrl Pts',(0.902193646979983,-0.237231147975234,
-1.3735491215176));
#21924=CARTESIAN_POINT('Ctrl Pts',(0.867957148219442,-0.166543350814306,
-1.39550172959303));
#21925=CARTESIAN_POINT('Ctrl Pts',(0.854205272175555,-0.123401821157026,
-1.40380622184538));
#21926=CARTESIAN_POINT('Ctrl Pts',(0.846804978391753,-0.0793800000000001,
-1.40825612658882));
#21927=CARTESIAN_POINT('Origin',(1.18440385848747,-0.07938,-1.18440385848747));
#21928=CARTESIAN_POINT('Origin',(0.,-0.27783,0.));
#21929=CARTESIAN_POINT('',(-1.643248,-0.47628,2.01239840340529E-16));
#21930=CARTESIAN_POINT('Origin',(0.,-0.47628,0.));
#21931=CARTESIAN_POINT('',(-1.643248,-0.27783,2.01239840340529E-16));
#21932=CARTESIAN_POINT('',(1.59456899932179,-0.07938,0.397005914195118));
#21933=CARTESIAN_POINT('Origin',(0.,-0.07938,0.));
#21934=CARTESIAN_POINT('',(1.59456899932179,-0.07938,-0.397005914195118));
#21935=CARTESIAN_POINT('Ctrl Pts',(1.59456899932179,-0.0793800000000001,
0.397005914195118));
#21936=CARTESIAN_POINT('Ctrl Pts',(1.59665523941937,-0.123401821157026,
0.388626558458099));
#21937=CARTESIAN_POINT('Ctrl Pts',(1.60050712143809,-0.166543350814306,
0.373030350867485));
#21938=CARTESIAN_POINT('Ctrl Pts',(1.60919314384089,-0.237231147975234,
0.333298652394954));
#21939=CARTESIAN_POINT('Ctrl Pts',(1.61365775139403,-0.266264900654909,
0.311480544243686));
#21940=CARTESIAN_POINT('Ctrl Pts',(1.62252828437015,-0.317195968905306,
0.261368388670537));
#21941=CARTESIAN_POINT('Ctrl Pts',(1.62691869420078,-0.33909093068465,0.233069203882014));
#21942=CARTESIAN_POINT('Ctrl Pts',(1.63426473152765,-0.373586846396559,
0.174042761838764));
#21943=CARTESIAN_POINT('Ctrl Pts',(1.63761964365402,-0.388086240756494,
0.140365781471549));
#21944=CARTESIAN_POINT('Ctrl Pts',(1.64212536811722,-0.407068917407805,
0.0701778381840612));
#21945=CARTESIAN_POINT('Ctrl Pts',(1.643248,-0.411552957311693,0.0336652739555916));
#21946=CARTESIAN_POINT('Ctrl Pts',(1.643248,-0.411552957311693,-0.0336652739555916));
#21947=CARTESIAN_POINT('Ctrl Pts',(1.64212536811722,-0.407068917407805,
-0.0701778381840612));
#21948=CARTESIAN_POINT('Ctrl Pts',(1.63761964365402,-0.388086240756494,
-0.140365781471549));
#21949=CARTESIAN_POINT('Ctrl Pts',(1.63426473152765,-0.373586846396559,
-0.174042761838764));
#21950=CARTESIAN_POINT('Ctrl Pts',(1.62691869420078,-0.33909093068465,-0.233069203882014));
#21951=CARTESIAN_POINT('Ctrl Pts',(1.62252828437015,-0.317195968905306,
-0.261368388670537));
#21952=CARTESIAN_POINT('Ctrl Pts',(1.61365775139403,-0.266264900654909,
-0.311480544243686));
#21953=CARTESIAN_POINT('Ctrl Pts',(1.60919314384089,-0.237231147975234,
-0.333298652394954));
#21954=CARTESIAN_POINT('Ctrl Pts',(1.60050712143809,-0.166543350814306,
-0.373030350867485));
#21955=CARTESIAN_POINT('Ctrl Pts',(1.59665523941937,-0.123401821157026,
-0.388626558458099));
#21956=CARTESIAN_POINT('Ctrl Pts',(1.59456899932179,-0.07938,-0.397005914195118));
#21957=CARTESIAN_POINT('Origin',(0.,-0.07938,0.));
#21958=CARTESIAN_POINT('Origin',(0.,-0.07938,0.));
#21959=CARTESIAN_POINT('Origin',(1.675,-0.07938,0.));
#21960=CARTESIAN_POINT('Origin',(1.675,0.,0.));
#21961=CARTESIAN_POINT('Origin',(1.675,-0.07938,0.));
#21962=CARTESIAN_POINT('Origin',(0.,-0.47628,0.));
#21963=CARTESIAN_POINT('Origin',(0.,-0.07938,0.));
#57820=UNCERTAINTY_MEASURE_WITH_UNIT(LENGTH_MEASURE(0.001),#57901,
'DISTANCE_ACCURACY_VALUE',
'Maximum model space distance between geometric entities at asserted c
onnectivities');
#57841=UNCERTAINTY_MEASURE_WITH_UNIT(LENGTH_MEASURE(0.001),#57901,
'DISTANCE_ACCURACY_VALUE',
'Maximum model space distance between geometric entities at asserted c
onnectivities');
#57879=(
GEOMETRIC_REPRESENTATION_CONTEXT(3)
GLOBAL_UNCERTAINTY_ASSIGNED_CONTEXT((#57820))
GLOBAL_UNIT_ASSIGNED_CONTEXT((#57901,#57903,#57904))
REPRESENTATION_CONTEXT('','3D')
);
#57900=(
GEOMETRIC_REPRESENTATION_CONTEXT(3)
GLOBAL_UNCERTAINTY_ASSIGNED_CONTEXT((#57841))
GLOBAL_UNIT_ASSIGNED_CONTEXT((#57901,#57903,#57904))
REPRESENTATION_CONTEXT('','3D')
);
#57901=(
LENGTH_UNIT()
NAMED_UNIT(*)
SI_UNIT(.CENTI.,.METRE.)
);
#57903=(
NAMED_UNIT(*)
PLANE_ANGLE_UNIT()
SI_UNIT($,.RADIAN.)
);
#57904=(
NAMED_UNIT(*)
SI_UNIT($,.STERADIAN.)
SOLID_ANGLE_UNIT()
);
#57942=SHAPE_DEFINITION_REPRESENTATION(#58008,#58146);
#58008=PRODUCT_DEFINITION_SHAPE('',$,#58205);
#58146=SHAPE_REPRESENTATION('',(#14965),#57879);
#58167=PRODUCT_DEFINITION_CONTEXT('part definition',#58343,'design');
#58205=PRODUCT_DEFINITION('Cage (1)','Cage (1)',#58263,#58167);
#58263=PRODUCT_DEFINITION_FORMATION('',$,#58382);
#58343=APPLICATION_CONTEXT(
'Core Data for Automotive Mechanical Design Process');
#58344=PRODUCT_CONTEXT('part definition',#58343,'mechanical');
#58382=PRODUCT('Cage (1)','Cage (1)','Cage (1)',(#58344));
#58459=COLOUR_RGB('Grey',0.48,0.52,0.57);
#58460=FILL_AREA_STYLE_COLOUR('',#58459);
#58461=FILL_AREA_STYLE('',(#58460));
#58462=SURFACE_STYLE_FILL_AREA(#58461);
#58463=SURFACE_SIDE_STYLE('',(#58462));
#58464=SURFACE_STYLE_USAGE(.BOTH.,#58463);
#58465=PRESENTATION_STYLE_ASSIGNMENT((#58464));
ENDSEC;
END-ISO-10303-21;
